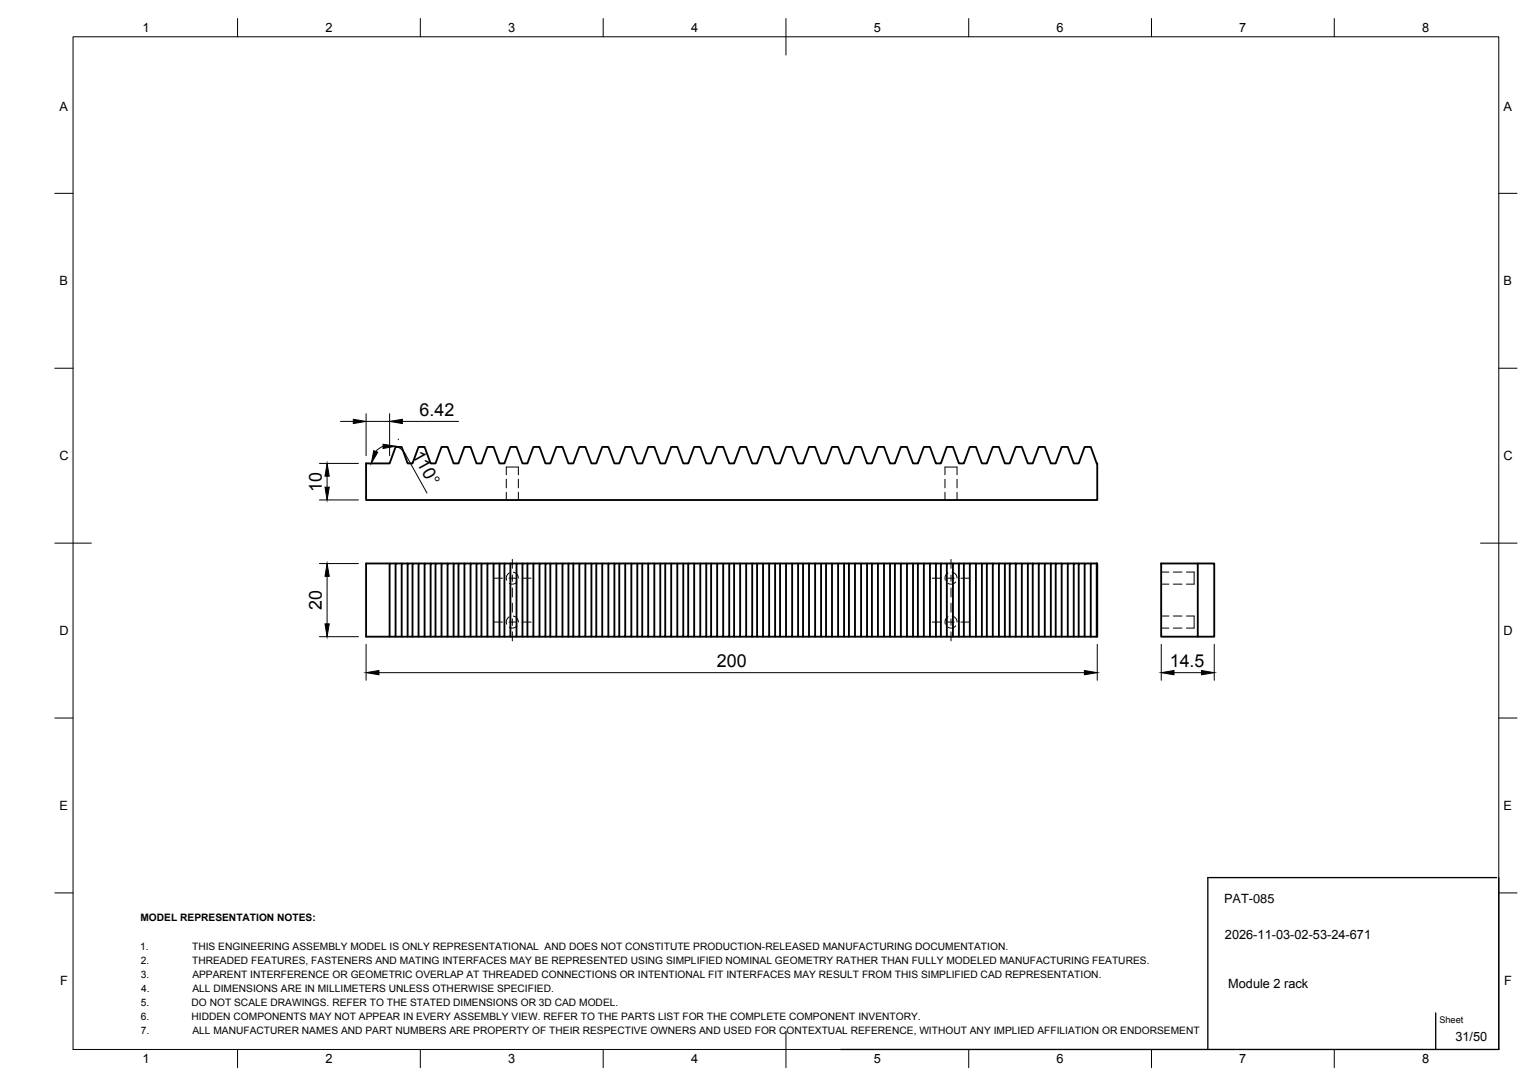
ISO-10303-21;
HEADER;
/* Generated by software containing ST-Developer
 * from STEP Tools, Inc. (www.steptools.com) 
 */

FILE_DESCRIPTION(
/* description */ ('Rack and pinion manual slide'),
/* implementation_level */ '2;1');

FILE_NAME(
/* name */ 'Module 2 rack.step',
/* time_stamp */ '2026-10-28T03:22:49-07:00',
/* author */ (''),
/* organization */ (''),
/* preprocessor_version */ 'ST-DEVELOPER v20.2',
/* originating_system */ 'Autodesk Translation Framework v15.17.0.0',
/* authorisation */ '');

FILE_SCHEMA (('AUTOMOTIVE_DESIGN { 1 0 10303 214 3 1 1 }'));
ENDSEC;

DATA;
#10=MECHANICAL_DESIGN_GEOMETRIC_PRESENTATION_REPRESENTATION('',(#765),#34851);
#666=SHAPE_REPRESENTATION_RELATIONSHIP('SRR','None',#35103,#712);
#712=ADVANCED_BREP_SHAPE_REPRESENTATION('',(#816),#34828);
#765=STYLED_ITEM('',(#35397),#816);
#816=MANIFOLD_SOLID_BREP('Body1',#13787);
#1001=FACE_BOUND('',#2793,.T.);
#1002=FACE_BOUND('',#2794,.T.);
#1003=FACE_BOUND('',#2795,.T.);
#1004=FACE_BOUND('',#2796,.T.);
#1251=PLANE('',#14966);
#1252=PLANE('',#14970);
#1253=PLANE('',#14974);
#1254=PLANE('',#14978);
#1255=PLANE('',#14979);
#1256=PLANE('',#14980);
#1257=PLANE('',#14981);
#1258=PLANE('',#14982);
#1259=PLANE('',#14983);
#1260=PLANE('',#14984);
#1261=PLANE('',#14985);
#1262=PLANE('',#14986);
#1263=PLANE('',#14987);
#1264=PLANE('',#14988);
#1265=PLANE('',#14989);
#1266=PLANE('',#14990);
#1267=PLANE('',#14991);
#1268=PLANE('',#14992);
#1269=PLANE('',#14993);
#1270=PLANE('',#14994);
#1271=PLANE('',#14995);
#1272=PLANE('',#14996);
#1273=PLANE('',#14997);
#1274=PLANE('',#14998);
#1275=PLANE('',#14999);
#1276=PLANE('',#15000);
#1277=PLANE('',#15001);
#1278=PLANE('',#15002);
#1279=PLANE('',#15003);
#1280=PLANE('',#15004);
#1281=PLANE('',#15005);
#1282=PLANE('',#15006);
#1283=PLANE('',#15007);
#1284=PLANE('',#15008);
#1285=PLANE('',#15009);
#1286=PLANE('',#15010);
#1287=PLANE('',#15011);
#1288=PLANE('',#15012);
#1289=PLANE('',#15013);
#1290=PLANE('',#15014);
#1291=PLANE('',#15015);
#1292=PLANE('',#15016);
#1293=PLANE('',#15017);
#1294=PLANE('',#15018);
#1295=PLANE('',#15019);
#1296=PLANE('',#15020);
#1297=PLANE('',#15021);
#1298=PLANE('',#15022);
#1299=PLANE('',#15023);
#1300=PLANE('',#15024);
#1301=PLANE('',#15025);
#1302=PLANE('',#15026);
#1303=PLANE('',#15027);
#1304=PLANE('',#15028);
#1305=PLANE('',#15029);
#1306=PLANE('',#15030);
#1307=PLANE('',#15031);
#1308=PLANE('',#15032);
#1309=PLANE('',#15033);
#1310=PLANE('',#15034);
#1311=PLANE('',#15035);
#1312=PLANE('',#15036);
#1313=PLANE('',#15037);
#1314=PLANE('',#15038);
#1315=PLANE('',#15039);
#1316=PLANE('',#15040);
#1317=PLANE('',#15041);
#1318=PLANE('',#15042);
#1319=PLANE('',#15043);
#1320=PLANE('',#15044);
#1321=PLANE('',#15045);
#1322=PLANE('',#15046);
#1323=PLANE('',#15047);
#1324=PLANE('',#15048);
#1325=PLANE('',#15049);
#1326=PLANE('',#15050);
#1327=PLANE('',#15051);
#1328=PLANE('',#15052);
#1329=PLANE('',#15053);
#1330=PLANE('',#15054);
#1331=PLANE('',#15055);
#1332=PLANE('',#15056);
#1333=PLANE('',#15057);
#1334=PLANE('',#15058);
#1335=PLANE('',#15059);
#1336=PLANE('',#15060);
#1337=PLANE('',#15061);
#1338=PLANE('',#15062);
#1339=PLANE('',#15063);
#1340=PLANE('',#15064);
#1341=PLANE('',#15065);
#1342=PLANE('',#15066);
#1343=PLANE('',#15067);
#1344=PLANE('',#15068);
#1345=PLANE('',#15069);
#1346=PLANE('',#15070);
#1347=PLANE('',#15071);
#1348=PLANE('',#15072);
#1349=PLANE('',#15073);
#1350=PLANE('',#15074);
#1351=PLANE('',#15075);
#1352=PLANE('',#15076);
#1353=PLANE('',#15077);
#1354=PLANE('',#15078);
#1355=PLANE('',#15079);
#1356=PLANE('',#15080);
#1357=PLANE('',#15081);
#1358=PLANE('',#15082);
#1359=PLANE('',#15083);
#1360=PLANE('',#15084);
#1361=PLANE('',#15085);
#1362=PLANE('',#15086);
#1363=PLANE('',#15087);
#1364=PLANE('',#15088);
#1365=PLANE('',#15089);
#1366=PLANE('',#15090);
#1367=PLANE('',#15091);
#1368=PLANE('',#15092);
#1369=PLANE('',#15093);
#1370=PLANE('',#15094);
#1371=PLANE('',#15095);
#1372=PLANE('',#15096);
#1373=PLANE('',#15097);
#1374=PLANE('',#15098);
#1375=PLANE('',#15099);
#1376=PLANE('',#15100);
#1377=PLANE('',#15101);
#1378=PLANE('',#15102);
#1379=PLANE('',#15103);
#1380=PLANE('',#15104);
#1381=PLANE('',#15105);
#1382=PLANE('',#15106);
#1383=PLANE('',#15107);
#1384=PLANE('',#15108);
#1876=FACE_OUTER_BOUND('',#2783,.T.);
#1877=FACE_OUTER_BOUND('',#2784,.T.);
#1878=FACE_OUTER_BOUND('',#2785,.T.);
#1879=FACE_OUTER_BOUND('',#2786,.T.);
#1880=FACE_OUTER_BOUND('',#2787,.T.);
#1881=FACE_OUTER_BOUND('',#2788,.T.);
#1882=FACE_OUTER_BOUND('',#2789,.T.);
#1883=FACE_OUTER_BOUND('',#2790,.T.);
#1884=FACE_OUTER_BOUND('',#2791,.T.);
#1885=FACE_OUTER_BOUND('',#2792,.T.);
#1886=FACE_OUTER_BOUND('',#2797,.T.);
#1887=FACE_OUTER_BOUND('',#2798,.T.);
#1888=FACE_OUTER_BOUND('',#2799,.T.);
#1889=FACE_OUTER_BOUND('',#2800,.T.);
#1890=FACE_OUTER_BOUND('',#2801,.T.);
#1891=FACE_OUTER_BOUND('',#2802,.T.);
#1892=FACE_OUTER_BOUND('',#2803,.T.);
#1893=FACE_OUTER_BOUND('',#2804,.T.);
#1894=FACE_OUTER_BOUND('',#2805,.T.);
#1895=FACE_OUTER_BOUND('',#2806,.T.);
#1896=FACE_OUTER_BOUND('',#2807,.T.);
#1897=FACE_OUTER_BOUND('',#2808,.T.);
#1898=FACE_OUTER_BOUND('',#2809,.T.);
#1899=FACE_OUTER_BOUND('',#2810,.T.);
#1900=FACE_OUTER_BOUND('',#2811,.T.);
#1901=FACE_OUTER_BOUND('',#2812,.T.);
#1902=FACE_OUTER_BOUND('',#2813,.T.);
#1903=FACE_OUTER_BOUND('',#2814,.T.);
#1904=FACE_OUTER_BOUND('',#2815,.T.);
#1905=FACE_OUTER_BOUND('',#2816,.T.);
#1906=FACE_OUTER_BOUND('',#2817,.T.);
#1907=FACE_OUTER_BOUND('',#2818,.T.);
#1908=FACE_OUTER_BOUND('',#2819,.T.);
#1909=FACE_OUTER_BOUND('',#2820,.T.);
#1910=FACE_OUTER_BOUND('',#2821,.T.);
#1911=FACE_OUTER_BOUND('',#2822,.T.);
#1912=FACE_OUTER_BOUND('',#2823,.T.);
#1913=FACE_OUTER_BOUND('',#2824,.T.);
#1914=FACE_OUTER_BOUND('',#2825,.T.);
#1915=FACE_OUTER_BOUND('',#2826,.T.);
#1916=FACE_OUTER_BOUND('',#2827,.T.);
#1917=FACE_OUTER_BOUND('',#2828,.T.);
#1918=FACE_OUTER_BOUND('',#2829,.T.);
#1919=FACE_OUTER_BOUND('',#2830,.T.);
#1920=FACE_OUTER_BOUND('',#2831,.T.);
#1921=FACE_OUTER_BOUND('',#2832,.T.);
#1922=FACE_OUTER_BOUND('',#2833,.T.);
#1923=FACE_OUTER_BOUND('',#2834,.T.);
#1924=FACE_OUTER_BOUND('',#2835,.T.);
#1925=FACE_OUTER_BOUND('',#2836,.T.);
#1926=FACE_OUTER_BOUND('',#2837,.T.);
#1927=FACE_OUTER_BOUND('',#2838,.T.);
#1928=FACE_OUTER_BOUND('',#2839,.T.);
#1929=FACE_OUTER_BOUND('',#2840,.T.);
#1930=FACE_OUTER_BOUND('',#2841,.T.);
#1931=FACE_OUTER_BOUND('',#2842,.T.);
#1932=FACE_OUTER_BOUND('',#2843,.T.);
#1933=FACE_OUTER_BOUND('',#2844,.T.);
#1934=FACE_OUTER_BOUND('',#2845,.T.);
#1935=FACE_OUTER_BOUND('',#2846,.T.);
#1936=FACE_OUTER_BOUND('',#2847,.T.);
#1937=FACE_OUTER_BOUND('',#2848,.T.);
#1938=FACE_OUTER_BOUND('',#2849,.T.);
#1939=FACE_OUTER_BOUND('',#2850,.T.);
#1940=FACE_OUTER_BOUND('',#2851,.T.);
#1941=FACE_OUTER_BOUND('',#2852,.T.);
#1942=FACE_OUTER_BOUND('',#2853,.T.);
#1943=FACE_OUTER_BOUND('',#2854,.T.);
#1944=FACE_OUTER_BOUND('',#2855,.T.);
#1945=FACE_OUTER_BOUND('',#2856,.T.);
#1946=FACE_OUTER_BOUND('',#2857,.T.);
#1947=FACE_OUTER_BOUND('',#2858,.T.);
#1948=FACE_OUTER_BOUND('',#2859,.T.);
#1949=FACE_OUTER_BOUND('',#2860,.T.);
#1950=FACE_OUTER_BOUND('',#2861,.T.);
#1951=FACE_OUTER_BOUND('',#2862,.T.);
#1952=FACE_OUTER_BOUND('',#2863,.T.);
#1953=FACE_OUTER_BOUND('',#2864,.T.);
#1954=FACE_OUTER_BOUND('',#2865,.T.);
#1955=FACE_OUTER_BOUND('',#2866,.T.);
#1956=FACE_OUTER_BOUND('',#2867,.T.);
#1957=FACE_OUTER_BOUND('',#2868,.T.);
#1958=FACE_OUTER_BOUND('',#2869,.T.);
#1959=FACE_OUTER_BOUND('',#2870,.T.);
#1960=FACE_OUTER_BOUND('',#2871,.T.);
#1961=FACE_OUTER_BOUND('',#2872,.T.);
#1962=FACE_OUTER_BOUND('',#2873,.T.);
#1963=FACE_OUTER_BOUND('',#2874,.T.);
#1964=FACE_OUTER_BOUND('',#2875,.T.);
#1965=FACE_OUTER_BOUND('',#2876,.T.);
#1966=FACE_OUTER_BOUND('',#2877,.T.);
#1967=FACE_OUTER_BOUND('',#2878,.T.);
#1968=FACE_OUTER_BOUND('',#2879,.T.);
#1969=FACE_OUTER_BOUND('',#2880,.T.);
#1970=FACE_OUTER_BOUND('',#2881,.T.);
#1971=FACE_OUTER_BOUND('',#2882,.T.);
#1972=FACE_OUTER_BOUND('',#2883,.T.);
#1973=FACE_OUTER_BOUND('',#2884,.T.);
#1974=FACE_OUTER_BOUND('',#2885,.T.);
#1975=FACE_OUTER_BOUND('',#2886,.T.);
#1976=FACE_OUTER_BOUND('',#2887,.T.);
#1977=FACE_OUTER_BOUND('',#2888,.T.);
#1978=FACE_OUTER_BOUND('',#2889,.T.);
#1979=FACE_OUTER_BOUND('',#2890,.T.);
#1980=FACE_OUTER_BOUND('',#2891,.T.);
#1981=FACE_OUTER_BOUND('',#2892,.T.);
#1982=FACE_OUTER_BOUND('',#2893,.T.);
#1983=FACE_OUTER_BOUND('',#2894,.T.);
#1984=FACE_OUTER_BOUND('',#2895,.T.);
#1985=FACE_OUTER_BOUND('',#2896,.T.);
#1986=FACE_OUTER_BOUND('',#2897,.T.);
#1987=FACE_OUTER_BOUND('',#2898,.T.);
#1988=FACE_OUTER_BOUND('',#2899,.T.);
#1989=FACE_OUTER_BOUND('',#2900,.T.);
#1990=FACE_OUTER_BOUND('',#2901,.T.);
#1991=FACE_OUTER_BOUND('',#2902,.T.);
#1992=FACE_OUTER_BOUND('',#2903,.T.);
#1993=FACE_OUTER_BOUND('',#2904,.T.);
#1994=FACE_OUTER_BOUND('',#2905,.T.);
#1995=FACE_OUTER_BOUND('',#2906,.T.);
#1996=FACE_OUTER_BOUND('',#2907,.T.);
#1997=FACE_OUTER_BOUND('',#2908,.T.);
#1998=FACE_OUTER_BOUND('',#2909,.T.);
#1999=FACE_OUTER_BOUND('',#2910,.T.);
#2000=FACE_OUTER_BOUND('',#2911,.T.);
#2001=FACE_OUTER_BOUND('',#2912,.T.);
#2002=FACE_OUTER_BOUND('',#2913,.T.);
#2003=FACE_OUTER_BOUND('',#2914,.T.);
#2004=FACE_OUTER_BOUND('',#2915,.T.);
#2005=FACE_OUTER_BOUND('',#2916,.T.);
#2006=FACE_OUTER_BOUND('',#2917,.T.);
#2007=FACE_OUTER_BOUND('',#2918,.T.);
#2008=FACE_OUTER_BOUND('',#2919,.T.);
#2009=FACE_OUTER_BOUND('',#2920,.T.);
#2010=FACE_OUTER_BOUND('',#2921,.T.);
#2011=FACE_OUTER_BOUND('',#2922,.T.);
#2012=FACE_OUTER_BOUND('',#2923,.T.);
#2013=FACE_OUTER_BOUND('',#2924,.T.);
#2783=EDGE_LOOP('',(#10820,#10821,#10822,#10823));
#2784=EDGE_LOOP('',(#10824));
#2785=EDGE_LOOP('',(#10825,#10826,#10827,#10828));
#2786=EDGE_LOOP('',(#10829));
#2787=EDGE_LOOP('',(#10830,#10831,#10832,#10833));
#2788=EDGE_LOOP('',(#10834));
#2789=EDGE_LOOP('',(#10835,#10836,#10837,#10838));
#2790=EDGE_LOOP('',(#10839));
#2791=EDGE_LOOP('',(#10840,#10841,#10842,#10843));
#2792=EDGE_LOOP('',(#10844,#10845,#10846,#10847));
#2793=EDGE_LOOP('',(#10848));
#2794=EDGE_LOOP('',(#10849));
#2795=EDGE_LOOP('',(#10850));
#2796=EDGE_LOOP('',(#10851));
#2797=EDGE_LOOP('',(#10852,#10853,#10854,#10855));
#2798=EDGE_LOOP('',(#10856,#10857,#10858,#10859));
#2799=EDGE_LOOP('',(#10860,#10861,#10862,#10863));
#2800=EDGE_LOOP('',(#10864,#10865,#10866,#10867));
#2801=EDGE_LOOP('',(#10868,#10869,#10870,#10871));
#2802=EDGE_LOOP('',(#10872,#10873,#10874,#10875));
#2803=EDGE_LOOP('',(#10876,#10877,#10878,#10879));
#2804=EDGE_LOOP('',(#10880,#10881,#10882,#10883));
#2805=EDGE_LOOP('',(#10884,#10885,#10886,#10887));
#2806=EDGE_LOOP('',(#10888,#10889,#10890,#10891));
#2807=EDGE_LOOP('',(#10892,#10893,#10894,#10895));
#2808=EDGE_LOOP('',(#10896,#10897,#10898,#10899));
#2809=EDGE_LOOP('',(#10900,#10901,#10902,#10903));
#2810=EDGE_LOOP('',(#10904,#10905,#10906,#10907));
#2811=EDGE_LOOP('',(#10908,#10909,#10910,#10911));
#2812=EDGE_LOOP('',(#10912,#10913,#10914,#10915));
#2813=EDGE_LOOP('',(#10916,#10917,#10918,#10919));
#2814=EDGE_LOOP('',(#10920,#10921,#10922,#10923));
#2815=EDGE_LOOP('',(#10924,#10925,#10926,#10927));
#2816=EDGE_LOOP('',(#10928,#10929,#10930,#10931));
#2817=EDGE_LOOP('',(#10932,#10933,#10934,#10935));
#2818=EDGE_LOOP('',(#10936,#10937,#10938,#10939));
#2819=EDGE_LOOP('',(#10940,#10941,#10942,#10943));
#2820=EDGE_LOOP('',(#10944,#10945,#10946,#10947));
#2821=EDGE_LOOP('',(#10948,#10949,#10950,#10951));
#2822=EDGE_LOOP('',(#10952,#10953,#10954,#10955));
#2823=EDGE_LOOP('',(#10956,#10957,#10958,#10959));
#2824=EDGE_LOOP('',(#10960,#10961,#10962,#10963));
#2825=EDGE_LOOP('',(#10964,#10965,#10966,#10967));
#2826=EDGE_LOOP('',(#10968,#10969,#10970,#10971));
#2827=EDGE_LOOP('',(#10972,#10973,#10974,#10975));
#2828=EDGE_LOOP('',(#10976,#10977,#10978,#10979));
#2829=EDGE_LOOP('',(#10980,#10981,#10982,#10983));
#2830=EDGE_LOOP('',(#10984,#10985,#10986,#10987));
#2831=EDGE_LOOP('',(#10988,#10989,#10990,#10991));
#2832=EDGE_LOOP('',(#10992,#10993,#10994,#10995));
#2833=EDGE_LOOP('',(#10996,#10997,#10998,#10999));
#2834=EDGE_LOOP('',(#11000,#11001,#11002,#11003));
#2835=EDGE_LOOP('',(#11004,#11005,#11006,#11007));
#2836=EDGE_LOOP('',(#11008,#11009,#11010,#11011));
#2837=EDGE_LOOP('',(#11012,#11013,#11014,#11015));
#2838=EDGE_LOOP('',(#11016,#11017,#11018,#11019));
#2839=EDGE_LOOP('',(#11020,#11021,#11022,#11023));
#2840=EDGE_LOOP('',(#11024,#11025,#11026,#11027));
#2841=EDGE_LOOP('',(#11028,#11029,#11030,#11031));
#2842=EDGE_LOOP('',(#11032,#11033,#11034,#11035));
#2843=EDGE_LOOP('',(#11036,#11037,#11038,#11039));
#2844=EDGE_LOOP('',(#11040,#11041,#11042,#11043));
#2845=EDGE_LOOP('',(#11044,#11045,#11046,#11047));
#2846=EDGE_LOOP('',(#11048,#11049,#11050,#11051));
#2847=EDGE_LOOP('',(#11052,#11053,#11054,#11055));
#2848=EDGE_LOOP('',(#11056,#11057,#11058,#11059));
#2849=EDGE_LOOP('',(#11060,#11061,#11062,#11063));
#2850=EDGE_LOOP('',(#11064,#11065,#11066,#11067));
#2851=EDGE_LOOP('',(#11068,#11069,#11070,#11071));
#2852=EDGE_LOOP('',(#11072,#11073,#11074,#11075));
#2853=EDGE_LOOP('',(#11076,#11077,#11078,#11079));
#2854=EDGE_LOOP('',(#11080,#11081,#11082,#11083));
#2855=EDGE_LOOP('',(#11084,#11085,#11086,#11087));
#2856=EDGE_LOOP('',(#11088,#11089,#11090,#11091));
#2857=EDGE_LOOP('',(#11092,#11093,#11094,#11095));
#2858=EDGE_LOOP('',(#11096,#11097,#11098,#11099));
#2859=EDGE_LOOP('',(#11100,#11101,#11102,#11103));
#2860=EDGE_LOOP('',(#11104,#11105,#11106,#11107));
#2861=EDGE_LOOP('',(#11108,#11109,#11110,#11111));
#2862=EDGE_LOOP('',(#11112,#11113,#11114,#11115));
#2863=EDGE_LOOP('',(#11116,#11117,#11118,#11119));
#2864=EDGE_LOOP('',(#11120,#11121,#11122,#11123));
#2865=EDGE_LOOP('',(#11124,#11125,#11126,#11127));
#2866=EDGE_LOOP('',(#11128,#11129,#11130,#11131));
#2867=EDGE_LOOP('',(#11132,#11133,#11134,#11135));
#2868=EDGE_LOOP('',(#11136,#11137,#11138,#11139));
#2869=EDGE_LOOP('',(#11140,#11141,#11142,#11143));
#2870=EDGE_LOOP('',(#11144,#11145,#11146,#11147));
#2871=EDGE_LOOP('',(#11148,#11149,#11150,#11151));
#2872=EDGE_LOOP('',(#11152,#11153,#11154,#11155));
#2873=EDGE_LOOP('',(#11156,#11157,#11158,#11159));
#2874=EDGE_LOOP('',(#11160,#11161,#11162,#11163));
#2875=EDGE_LOOP('',(#11164,#11165,#11166,#11167));
#2876=EDGE_LOOP('',(#11168,#11169,#11170,#11171));
#2877=EDGE_LOOP('',(#11172,#11173,#11174,#11175));
#2878=EDGE_LOOP('',(#11176,#11177,#11178,#11179));
#2879=EDGE_LOOP('',(#11180,#11181,#11182,#11183));
#2880=EDGE_LOOP('',(#11184,#11185,#11186,#11187));
#2881=EDGE_LOOP('',(#11188,#11189,#11190,#11191));
#2882=EDGE_LOOP('',(#11192,#11193,#11194,#11195));
#2883=EDGE_LOOP('',(#11196,#11197,#11198,#11199));
#2884=EDGE_LOOP('',(#11200,#11201,#11202,#11203));
#2885=EDGE_LOOP('',(#11204,#11205,#11206,#11207));
#2886=EDGE_LOOP('',(#11208,#11209,#11210,#11211));
#2887=EDGE_LOOP('',(#11212,#11213,#11214,#11215));
#2888=EDGE_LOOP('',(#11216,#11217,#11218,#11219));
#2889=EDGE_LOOP('',(#11220,#11221,#11222,#11223));
#2890=EDGE_LOOP('',(#11224,#11225,#11226,#11227));
#2891=EDGE_LOOP('',(#11228,#11229,#11230,#11231));
#2892=EDGE_LOOP('',(#11232,#11233,#11234,#11235));
#2893=EDGE_LOOP('',(#11236,#11237,#11238,#11239));
#2894=EDGE_LOOP('',(#11240,#11241,#11242,#11243));
#2895=EDGE_LOOP('',(#11244,#11245,#11246,#11247));
#2896=EDGE_LOOP('',(#11248,#11249,#11250,#11251));
#2897=EDGE_LOOP('',(#11252,#11253,#11254,#11255));
#2898=EDGE_LOOP('',(#11256,#11257,#11258,#11259));
#2899=EDGE_LOOP('',(#11260,#11261,#11262,#11263));
#2900=EDGE_LOOP('',(#11264,#11265,#11266,#11267));
#2901=EDGE_LOOP('',(#11268,#11269,#11270,#11271));
#2902=EDGE_LOOP('',(#11272,#11273,#11274,#11275));
#2903=EDGE_LOOP('',(#11276,#11277,#11278,#11279));
#2904=EDGE_LOOP('',(#11280,#11281,#11282,#11283));
#2905=EDGE_LOOP('',(#11284,#11285,#11286,#11287));
#2906=EDGE_LOOP('',(#11288,#11289,#11290,#11291));
#2907=EDGE_LOOP('',(#11292,#11293,#11294,#11295));
#2908=EDGE_LOOP('',(#11296,#11297,#11298,#11299));
#2909=EDGE_LOOP('',(#11300,#11301,#11302,#11303));
#2910=EDGE_LOOP('',(#11304,#11305,#11306,#11307));
#2911=EDGE_LOOP('',(#11308,#11309,#11310,#11311));
#2912=EDGE_LOOP('',(#11312,#11313,#11314,#11315));
#2913=EDGE_LOOP('',(#11316,#11317,#11318,#11319));
#2914=EDGE_LOOP('',(#11320,#11321,#11322,#11323));
#2915=EDGE_LOOP('',(#11324,#11325,#11326,#11327));
#2916=EDGE_LOOP('',(#11328,#11329,#11330,#11331));
#2917=EDGE_LOOP('',(#11332,#11333,#11334,#11335));
#2918=EDGE_LOOP('',(#11336,#11337,#11338,#11339));
#2919=EDGE_LOOP('',(#11340,#11341,#11342,#11343));
#2920=EDGE_LOOP('',(#11344,#11345,#11346,#11347));
#2921=EDGE_LOOP('',(#11348,#11349,#11350,#11351));
#2922=EDGE_LOOP('',(#11352,#11353,#11354,#11355));
#2923=EDGE_LOOP('',(#11356,#11357,#11358,#11359,#11360,#11361,#11362,#11363,
#11364,#11365,#11366,#11367,#11368,#11369,#11370,#11371,#11372,#11373,#11374,
#11375,#11376,#11377,#11378,#11379,#11380,#11381,#11382,#11383,#11384,#11385,
#11386,#11387,#11388,#11389,#11390,#11391,#11392,#11393,#11394,#11395,#11396,
#11397,#11398,#11399,#11400,#11401,#11402,#11403,#11404,#11405,#11406,#11407,
#11408,#11409,#11410,#11411,#11412,#11413,#11414,#11415,#11416,#11417,#11418,
#11419,#11420,#11421,#11422,#11423,#11424,#11425,#11426,#11427,#11428,#11429,
#11430,#11431,#11432,#11433,#11434,#11435,#11436,#11437,#11438,#11439,#11440,
#11441,#11442,#11443,#11444,#11445,#11446,#11447,#11448,#11449,#11450,#11451,
#11452,#11453,#11454,#11455,#11456,#11457,#11458,#11459,#11460,#11461,#11462,
#11463,#11464,#11465,#11466,#11467,#11468,#11469,#11470,#11471,#11472,#11473,
#11474,#11475,#11476,#11477,#11478,#11479,#11480,#11481,#11482,#11483));
#2924=EDGE_LOOP('',(#11484,#11485,#11486,#11487,#11488,#11489,#11490,#11491,
#11492,#11493,#11494,#11495,#11496,#11497,#11498,#11499,#11500,#11501,#11502,
#11503,#11504,#11505,#11506,#11507,#11508,#11509,#11510,#11511,#11512,#11513,
#11514,#11515,#11516,#11517,#11518,#11519,#11520,#11521,#11522,#11523,#11524,
#11525,#11526,#11527,#11528,#11529,#11530,#11531,#11532,#11533,#11534,#11535,
#11536,#11537,#11538,#11539,#11540,#11541,#11542,#11543,#11544,#11545,#11546,
#11547,#11548,#11549,#11550,#11551,#11552,#11553,#11554,#11555,#11556,#11557,
#11558,#11559,#11560,#11561,#11562,#11563,#11564,#11565,#11566,#11567,#11568,
#11569,#11570,#11571,#11572,#11573,#11574,#11575,#11576,#11577,#11578,#11579,
#11580,#11581,#11582,#11583,#11584,#11585,#11586,#11587,#11588,#11589,#11590,
#11591,#11592,#11593,#11594,#11595,#11596,#11597,#11598,#11599,#11600,#11601,
#11602,#11603,#11604,#11605,#11606,#11607,#11608,#11609,#11610,#11611));
#3734=LINE('',#21459,#5025);
#3735=LINE('',#21466,#5026);
#3736=LINE('',#21473,#5027);
#3737=LINE('',#21480,#5028);
#3738=LINE('',#21486,#5029);
#3739=LINE('',#21488,#5030);
#3740=LINE('',#21490,#5031);
#3741=LINE('',#21491,#5032);
#3742=LINE('',#21494,#5033);
#3743=LINE('',#21496,#5034);
#3744=LINE('',#21497,#5035);
#3745=LINE('',#21500,#5036);
#3746=LINE('',#21502,#5037);
#3747=LINE('',#21503,#5038);
#3748=LINE('',#21506,#5039);
#3749=LINE('',#21508,#5040);
#3750=LINE('',#21509,#5041);
#3751=LINE('',#21512,#5042);
#3752=LINE('',#21514,#5043);
#3753=LINE('',#21515,#5044);
#3754=LINE('',#21518,#5045);
#3755=LINE('',#21520,#5046);
#3756=LINE('',#21521,#5047);
#3757=LINE('',#21524,#5048);
#3758=LINE('',#21526,#5049);
#3759=LINE('',#21527,#5050);
#3760=LINE('',#21530,#5051);
#3761=LINE('',#21532,#5052);
#3762=LINE('',#21533,#5053);
#3763=LINE('',#21536,#5054);
#3764=LINE('',#21538,#5055);
#3765=LINE('',#21539,#5056);
#3766=LINE('',#21542,#5057);
#3767=LINE('',#21544,#5058);
#3768=LINE('',#21545,#5059);
#3769=LINE('',#21548,#5060);
#3770=LINE('',#21550,#5061);
#3771=LINE('',#21551,#5062);
#3772=LINE('',#21554,#5063);
#3773=LINE('',#21556,#5064);
#3774=LINE('',#21557,#5065);
#3775=LINE('',#21560,#5066);
#3776=LINE('',#21562,#5067);
#3777=LINE('',#21563,#5068);
#3778=LINE('',#21566,#5069);
#3779=LINE('',#21568,#5070);
#3780=LINE('',#21569,#5071);
#3781=LINE('',#21572,#5072);
#3782=LINE('',#21574,#5073);
#3783=LINE('',#21575,#5074);
#3784=LINE('',#21578,#5075);
#3785=LINE('',#21580,#5076);
#3786=LINE('',#21581,#5077);
#3787=LINE('',#21584,#5078);
#3788=LINE('',#21586,#5079);
#3789=LINE('',#21587,#5080);
#3790=LINE('',#21590,#5081);
#3791=LINE('',#21592,#5082);
#3792=LINE('',#21593,#5083);
#3793=LINE('',#21596,#5084);
#3794=LINE('',#21598,#5085);
#3795=LINE('',#21599,#5086);
#3796=LINE('',#21602,#5087);
#3797=LINE('',#21604,#5088);
#3798=LINE('',#21605,#5089);
#3799=LINE('',#21608,#5090);
#3800=LINE('',#21610,#5091);
#3801=LINE('',#21611,#5092);
#3802=LINE('',#21614,#5093);
#3803=LINE('',#21616,#5094);
#3804=LINE('',#21617,#5095);
#3805=LINE('',#21620,#5096);
#3806=LINE('',#21622,#5097);
#3807=LINE('',#21623,#5098);
#3808=LINE('',#21626,#5099);
#3809=LINE('',#21628,#5100);
#3810=LINE('',#21629,#5101);
#3811=LINE('',#21632,#5102);
#3812=LINE('',#21634,#5103);
#3813=LINE('',#21635,#5104);
#3814=LINE('',#21638,#5105);
#3815=LINE('',#21640,#5106);
#3816=LINE('',#21641,#5107);
#3817=LINE('',#21644,#5108);
#3818=LINE('',#21646,#5109);
#3819=LINE('',#21647,#5110);
#3820=LINE('',#21650,#5111);
#3821=LINE('',#21652,#5112);
#3822=LINE('',#21653,#5113);
#3823=LINE('',#21656,#5114);
#3824=LINE('',#21658,#5115);
#3825=LINE('',#21659,#5116);
#3826=LINE('',#21662,#5117);
#3827=LINE('',#21664,#5118);
#3828=LINE('',#21665,#5119);
#3829=LINE('',#21668,#5120);
#3830=LINE('',#21670,#5121);
#3831=LINE('',#21671,#5122);
#3832=LINE('',#21674,#5123);
#3833=LINE('',#21676,#5124);
#3834=LINE('',#21677,#5125);
#3835=LINE('',#21680,#5126);
#3836=LINE('',#21682,#5127);
#3837=LINE('',#21683,#5128);
#3838=LINE('',#21686,#5129);
#3839=LINE('',#21688,#5130);
#3840=LINE('',#21689,#5131);
#3841=LINE('',#21692,#5132);
#3842=LINE('',#21694,#5133);
#3843=LINE('',#21695,#5134);
#3844=LINE('',#21698,#5135);
#3845=LINE('',#21700,#5136);
#3846=LINE('',#21701,#5137);
#3847=LINE('',#21704,#5138);
#3848=LINE('',#21706,#5139);
#3849=LINE('',#21707,#5140);
#3850=LINE('',#21710,#5141);
#3851=LINE('',#21712,#5142);
#3852=LINE('',#21713,#5143);
#3853=LINE('',#21716,#5144);
#3854=LINE('',#21718,#5145);
#3855=LINE('',#21719,#5146);
#3856=LINE('',#21722,#5147);
#3857=LINE('',#21724,#5148);
#3858=LINE('',#21725,#5149);
#3859=LINE('',#21728,#5150);
#3860=LINE('',#21730,#5151);
#3861=LINE('',#21731,#5152);
#3862=LINE('',#21734,#5153);
#3863=LINE('',#21736,#5154);
#3864=LINE('',#21737,#5155);
#3865=LINE('',#21740,#5156);
#3866=LINE('',#21742,#5157);
#3867=LINE('',#21743,#5158);
#3868=LINE('',#21746,#5159);
#3869=LINE('',#21748,#5160);
#3870=LINE('',#21749,#5161);
#3871=LINE('',#21752,#5162);
#3872=LINE('',#21754,#5163);
#3873=LINE('',#21755,#5164);
#3874=LINE('',#21758,#5165);
#3875=LINE('',#21760,#5166);
#3876=LINE('',#21761,#5167);
#3877=LINE('',#21764,#5168);
#3878=LINE('',#21766,#5169);
#3879=LINE('',#21767,#5170);
#3880=LINE('',#21770,#5171);
#3881=LINE('',#21772,#5172);
#3882=LINE('',#21773,#5173);
#3883=LINE('',#21776,#5174);
#3884=LINE('',#21778,#5175);
#3885=LINE('',#21779,#5176);
#3886=LINE('',#21782,#5177);
#3887=LINE('',#21784,#5178);
#3888=LINE('',#21785,#5179);
#3889=LINE('',#21788,#5180);
#3890=LINE('',#21790,#5181);
#3891=LINE('',#21791,#5182);
#3892=LINE('',#21794,#5183);
#3893=LINE('',#21796,#5184);
#3894=LINE('',#21797,#5185);
#3895=LINE('',#21800,#5186);
#3896=LINE('',#21802,#5187);
#3897=LINE('',#21803,#5188);
#3898=LINE('',#21806,#5189);
#3899=LINE('',#21808,#5190);
#3900=LINE('',#21809,#5191);
#3901=LINE('',#21812,#5192);
#3902=LINE('',#21814,#5193);
#3903=LINE('',#21815,#5194);
#3904=LINE('',#21818,#5195);
#3905=LINE('',#21820,#5196);
#3906=LINE('',#21821,#5197);
#3907=LINE('',#21824,#5198);
#3908=LINE('',#21826,#5199);
#3909=LINE('',#21827,#5200);
#3910=LINE('',#21830,#5201);
#3911=LINE('',#21832,#5202);
#3912=LINE('',#21833,#5203);
#3913=LINE('',#21836,#5204);
#3914=LINE('',#21838,#5205);
#3915=LINE('',#21839,#5206);
#3916=LINE('',#21842,#5207);
#3917=LINE('',#21844,#5208);
#3918=LINE('',#21845,#5209);
#3919=LINE('',#21848,#5210);
#3920=LINE('',#21850,#5211);
#3921=LINE('',#21851,#5212);
#3922=LINE('',#21854,#5213);
#3923=LINE('',#21856,#5214);
#3924=LINE('',#21857,#5215);
#3925=LINE('',#21860,#5216);
#3926=LINE('',#21862,#5217);
#3927=LINE('',#21863,#5218);
#3928=LINE('',#21866,#5219);
#3929=LINE('',#21868,#5220);
#3930=LINE('',#21869,#5221);
#3931=LINE('',#21872,#5222);
#3932=LINE('',#21874,#5223);
#3933=LINE('',#21875,#5224);
#3934=LINE('',#21878,#5225);
#3935=LINE('',#21880,#5226);
#3936=LINE('',#21881,#5227);
#3937=LINE('',#21884,#5228);
#3938=LINE('',#21886,#5229);
#3939=LINE('',#21887,#5230);
#3940=LINE('',#21890,#5231);
#3941=LINE('',#21892,#5232);
#3942=LINE('',#21893,#5233);
#3943=LINE('',#21896,#5234);
#3944=LINE('',#21898,#5235);
#3945=LINE('',#21899,#5236);
#3946=LINE('',#21902,#5237);
#3947=LINE('',#21904,#5238);
#3948=LINE('',#21905,#5239);
#3949=LINE('',#21908,#5240);
#3950=LINE('',#21910,#5241);
#3951=LINE('',#21911,#5242);
#3952=LINE('',#21914,#5243);
#3953=LINE('',#21916,#5244);
#3954=LINE('',#21917,#5245);
#3955=LINE('',#21920,#5246);
#3956=LINE('',#21922,#5247);
#3957=LINE('',#21923,#5248);
#3958=LINE('',#21926,#5249);
#3959=LINE('',#21928,#5250);
#3960=LINE('',#21929,#5251);
#3961=LINE('',#21932,#5252);
#3962=LINE('',#21934,#5253);
#3963=LINE('',#21935,#5254);
#3964=LINE('',#21938,#5255);
#3965=LINE('',#21940,#5256);
#3966=LINE('',#21941,#5257);
#3967=LINE('',#21944,#5258);
#3968=LINE('',#21946,#5259);
#3969=LINE('',#21947,#5260);
#3970=LINE('',#21950,#5261);
#3971=LINE('',#21952,#5262);
#3972=LINE('',#21953,#5263);
#3973=LINE('',#21956,#5264);
#3974=LINE('',#21958,#5265);
#3975=LINE('',#21959,#5266);
#3976=LINE('',#21962,#5267);
#3977=LINE('',#21964,#5268);
#3978=LINE('',#21965,#5269);
#3979=LINE('',#21968,#5270);
#3980=LINE('',#21970,#5271);
#3981=LINE('',#21971,#5272);
#3982=LINE('',#21974,#5273);
#3983=LINE('',#21976,#5274);
#3984=LINE('',#21977,#5275);
#3985=LINE('',#21980,#5276);
#3986=LINE('',#21982,#5277);
#3987=LINE('',#21983,#5278);
#3988=LINE('',#21986,#5279);
#3989=LINE('',#21988,#5280);
#3990=LINE('',#21989,#5281);
#3991=LINE('',#21992,#5282);
#3992=LINE('',#21994,#5283);
#3993=LINE('',#21995,#5284);
#3994=LINE('',#21998,#5285);
#3995=LINE('',#22000,#5286);
#3996=LINE('',#22001,#5287);
#3997=LINE('',#22004,#5288);
#3998=LINE('',#22006,#5289);
#3999=LINE('',#22007,#5290);
#4000=LINE('',#22010,#5291);
#4001=LINE('',#22012,#5292);
#4002=LINE('',#22013,#5293);
#4003=LINE('',#22016,#5294);
#4004=LINE('',#22018,#5295);
#4005=LINE('',#22019,#5296);
#4006=LINE('',#22022,#5297);
#4007=LINE('',#22024,#5298);
#4008=LINE('',#22025,#5299);
#4009=LINE('',#22028,#5300);
#4010=LINE('',#22030,#5301);
#4011=LINE('',#22031,#5302);
#4012=LINE('',#22034,#5303);
#4013=LINE('',#22036,#5304);
#4014=LINE('',#22037,#5305);
#4015=LINE('',#22040,#5306);
#4016=LINE('',#22042,#5307);
#4017=LINE('',#22043,#5308);
#4018=LINE('',#22046,#5309);
#4019=LINE('',#22048,#5310);
#4020=LINE('',#22049,#5311);
#4021=LINE('',#22052,#5312);
#4022=LINE('',#22054,#5313);
#4023=LINE('',#22055,#5314);
#4024=LINE('',#22058,#5315);
#4025=LINE('',#22060,#5316);
#4026=LINE('',#22061,#5317);
#4027=LINE('',#22064,#5318);
#4028=LINE('',#22066,#5319);
#4029=LINE('',#22067,#5320);
#4030=LINE('',#22070,#5321);
#4031=LINE('',#22072,#5322);
#4032=LINE('',#22073,#5323);
#4033=LINE('',#22076,#5324);
#4034=LINE('',#22078,#5325);
#4035=LINE('',#22079,#5326);
#4036=LINE('',#22082,#5327);
#4037=LINE('',#22084,#5328);
#4038=LINE('',#22085,#5329);
#4039=LINE('',#22088,#5330);
#4040=LINE('',#22090,#5331);
#4041=LINE('',#22091,#5332);
#4042=LINE('',#22094,#5333);
#4043=LINE('',#22096,#5334);
#4044=LINE('',#22097,#5335);
#4045=LINE('',#22100,#5336);
#4046=LINE('',#22102,#5337);
#4047=LINE('',#22103,#5338);
#4048=LINE('',#22106,#5339);
#4049=LINE('',#22108,#5340);
#4050=LINE('',#22109,#5341);
#4051=LINE('',#22112,#5342);
#4052=LINE('',#22114,#5343);
#4053=LINE('',#22115,#5344);
#4054=LINE('',#22118,#5345);
#4055=LINE('',#22120,#5346);
#4056=LINE('',#22121,#5347);
#4057=LINE('',#22124,#5348);
#4058=LINE('',#22126,#5349);
#4059=LINE('',#22127,#5350);
#4060=LINE('',#22130,#5351);
#4061=LINE('',#22132,#5352);
#4062=LINE('',#22133,#5353);
#4063=LINE('',#22136,#5354);
#4064=LINE('',#22138,#5355);
#4065=LINE('',#22139,#5356);
#4066=LINE('',#22142,#5357);
#4067=LINE('',#22144,#5358);
#4068=LINE('',#22145,#5359);
#4069=LINE('',#22148,#5360);
#4070=LINE('',#22150,#5361);
#4071=LINE('',#22151,#5362);
#4072=LINE('',#22154,#5363);
#4073=LINE('',#22156,#5364);
#4074=LINE('',#22157,#5365);
#4075=LINE('',#22160,#5366);
#4076=LINE('',#22162,#5367);
#4077=LINE('',#22163,#5368);
#4078=LINE('',#22166,#5369);
#4079=LINE('',#22168,#5370);
#4080=LINE('',#22169,#5371);
#4081=LINE('',#22172,#5372);
#4082=LINE('',#22174,#5373);
#4083=LINE('',#22175,#5374);
#4084=LINE('',#22178,#5375);
#4085=LINE('',#22180,#5376);
#4086=LINE('',#22181,#5377);
#4087=LINE('',#22184,#5378);
#4088=LINE('',#22186,#5379);
#4089=LINE('',#22187,#5380);
#4090=LINE('',#22190,#5381);
#4091=LINE('',#22192,#5382);
#4092=LINE('',#22193,#5383);
#4093=LINE('',#22196,#5384);
#4094=LINE('',#22198,#5385);
#4095=LINE('',#22199,#5386);
#4096=LINE('',#22202,#5387);
#4097=LINE('',#22204,#5388);
#4098=LINE('',#22205,#5389);
#4099=LINE('',#22208,#5390);
#4100=LINE('',#22210,#5391);
#4101=LINE('',#22211,#5392);
#4102=LINE('',#22214,#5393);
#4103=LINE('',#22216,#5394);
#4104=LINE('',#22217,#5395);
#4105=LINE('',#22220,#5396);
#4106=LINE('',#22222,#5397);
#4107=LINE('',#22223,#5398);
#4108=LINE('',#22226,#5399);
#4109=LINE('',#22228,#5400);
#4110=LINE('',#22229,#5401);
#4111=LINE('',#22232,#5402);
#4112=LINE('',#22234,#5403);
#4113=LINE('',#22235,#5404);
#4114=LINE('',#22238,#5405);
#4115=LINE('',#22240,#5406);
#4116=LINE('',#22241,#5407);
#4117=LINE('',#22244,#5408);
#4118=LINE('',#22246,#5409);
#4119=LINE('',#22247,#5410);
#4120=LINE('',#22249,#5411);
#4121=LINE('',#22250,#5412);
#5025=VECTOR('',#17406,0.164999999999999);
#5026=VECTOR('',#17415,0.165);
#5027=VECTOR('',#17424,0.165);
#5028=VECTOR('',#17433,0.164999999999999);
#5029=VECTOR('',#17440,1.);
#5030=VECTOR('',#17441,1.);
#5031=VECTOR('',#17442,1.);
#5032=VECTOR('',#17443,1.);
#5033=VECTOR('',#17446,1.);
#5034=VECTOR('',#17447,1.);
#5035=VECTOR('',#17448,1.);
#5036=VECTOR('',#17451,1.);
#5037=VECTOR('',#17452,1.);
#5038=VECTOR('',#17453,1.);
#5039=VECTOR('',#17456,1.);
#5040=VECTOR('',#17457,1.);
#5041=VECTOR('',#17458,1.);
#5042=VECTOR('',#17461,1.);
#5043=VECTOR('',#17462,1.);
#5044=VECTOR('',#17463,1.);
#5045=VECTOR('',#17466,1.);
#5046=VECTOR('',#17467,1.);
#5047=VECTOR('',#17468,1.);
#5048=VECTOR('',#17471,1.);
#5049=VECTOR('',#17472,1.);
#5050=VECTOR('',#17473,1.);
#5051=VECTOR('',#17476,1.);
#5052=VECTOR('',#17477,1.);
#5053=VECTOR('',#17478,1.);
#5054=VECTOR('',#17481,1.);
#5055=VECTOR('',#17482,1.);
#5056=VECTOR('',#17483,1.);
#5057=VECTOR('',#17486,1.);
#5058=VECTOR('',#17487,1.);
#5059=VECTOR('',#17488,1.);
#5060=VECTOR('',#17491,1.);
#5061=VECTOR('',#17492,1.);
#5062=VECTOR('',#17493,1.);
#5063=VECTOR('',#17496,1.);
#5064=VECTOR('',#17497,1.);
#5065=VECTOR('',#17498,1.);
#5066=VECTOR('',#17501,1.);
#5067=VECTOR('',#17502,1.);
#5068=VECTOR('',#17503,1.);
#5069=VECTOR('',#17506,1.);
#5070=VECTOR('',#17507,1.);
#5071=VECTOR('',#17508,1.);
#5072=VECTOR('',#17511,1.);
#5073=VECTOR('',#17512,1.);
#5074=VECTOR('',#17513,1.);
#5075=VECTOR('',#17516,1.);
#5076=VECTOR('',#17517,1.);
#5077=VECTOR('',#17518,1.);
#5078=VECTOR('',#17521,1.);
#5079=VECTOR('',#17522,1.);
#5080=VECTOR('',#17523,1.);
#5081=VECTOR('',#17526,1.);
#5082=VECTOR('',#17527,1.);
#5083=VECTOR('',#17528,1.);
#5084=VECTOR('',#17531,1.);
#5085=VECTOR('',#17532,1.);
#5086=VECTOR('',#17533,1.);
#5087=VECTOR('',#17536,1.);
#5088=VECTOR('',#17537,1.);
#5089=VECTOR('',#17538,1.);
#5090=VECTOR('',#17541,1.);
#5091=VECTOR('',#17542,1.);
#5092=VECTOR('',#17543,1.);
#5093=VECTOR('',#17546,1.);
#5094=VECTOR('',#17547,1.);
#5095=VECTOR('',#17548,1.);
#5096=VECTOR('',#17551,1.);
#5097=VECTOR('',#17552,1.);
#5098=VECTOR('',#17553,1.);
#5099=VECTOR('',#17556,1.);
#5100=VECTOR('',#17557,1.);
#5101=VECTOR('',#17558,1.);
#5102=VECTOR('',#17561,1.);
#5103=VECTOR('',#17562,1.);
#5104=VECTOR('',#17563,1.);
#5105=VECTOR('',#17566,1.);
#5106=VECTOR('',#17567,1.);
#5107=VECTOR('',#17568,1.);
#5108=VECTOR('',#17571,1.);
#5109=VECTOR('',#17572,1.);
#5110=VECTOR('',#17573,1.);
#5111=VECTOR('',#17576,1.);
#5112=VECTOR('',#17577,1.);
#5113=VECTOR('',#17578,1.);
#5114=VECTOR('',#17581,1.);
#5115=VECTOR('',#17582,1.);
#5116=VECTOR('',#17583,1.);
#5117=VECTOR('',#17586,1.);
#5118=VECTOR('',#17587,1.);
#5119=VECTOR('',#17588,1.);
#5120=VECTOR('',#17591,1.);
#5121=VECTOR('',#17592,1.);
#5122=VECTOR('',#17593,1.);
#5123=VECTOR('',#17596,1.);
#5124=VECTOR('',#17597,1.);
#5125=VECTOR('',#17598,1.);
#5126=VECTOR('',#17601,1.);
#5127=VECTOR('',#17602,1.);
#5128=VECTOR('',#17603,1.);
#5129=VECTOR('',#17606,1.);
#5130=VECTOR('',#17607,1.);
#5131=VECTOR('',#17608,1.);
#5132=VECTOR('',#17611,1.);
#5133=VECTOR('',#17612,1.);
#5134=VECTOR('',#17613,1.);
#5135=VECTOR('',#17616,1.);
#5136=VECTOR('',#17617,1.);
#5137=VECTOR('',#17618,1.);
#5138=VECTOR('',#17621,1.);
#5139=VECTOR('',#17622,1.);
#5140=VECTOR('',#17623,1.);
#5141=VECTOR('',#17626,1.);
#5142=VECTOR('',#17627,1.);
#5143=VECTOR('',#17628,1.);
#5144=VECTOR('',#17631,1.);
#5145=VECTOR('',#17632,1.);
#5146=VECTOR('',#17633,1.);
#5147=VECTOR('',#17636,1.);
#5148=VECTOR('',#17637,1.);
#5149=VECTOR('',#17638,1.);
#5150=VECTOR('',#17641,1.);
#5151=VECTOR('',#17642,1.);
#5152=VECTOR('',#17643,1.);
#5153=VECTOR('',#17646,1.);
#5154=VECTOR('',#17647,1.);
#5155=VECTOR('',#17648,1.);
#5156=VECTOR('',#17651,1.);
#5157=VECTOR('',#17652,1.);
#5158=VECTOR('',#17653,1.);
#5159=VECTOR('',#17656,1.);
#5160=VECTOR('',#17657,1.);
#5161=VECTOR('',#17658,1.);
#5162=VECTOR('',#17661,1.);
#5163=VECTOR('',#17662,1.);
#5164=VECTOR('',#17663,1.);
#5165=VECTOR('',#17666,1.);
#5166=VECTOR('',#17667,1.);
#5167=VECTOR('',#17668,1.);
#5168=VECTOR('',#17671,1.);
#5169=VECTOR('',#17672,1.);
#5170=VECTOR('',#17673,1.);
#5171=VECTOR('',#17676,1.);
#5172=VECTOR('',#17677,1.);
#5173=VECTOR('',#17678,1.);
#5174=VECTOR('',#17681,1.);
#5175=VECTOR('',#17682,1.);
#5176=VECTOR('',#17683,1.);
#5177=VECTOR('',#17686,1.);
#5178=VECTOR('',#17687,1.);
#5179=VECTOR('',#17688,1.);
#5180=VECTOR('',#17691,1.);
#5181=VECTOR('',#17692,1.);
#5182=VECTOR('',#17693,1.);
#5183=VECTOR('',#17696,1.);
#5184=VECTOR('',#17697,1.);
#5185=VECTOR('',#17698,1.);
#5186=VECTOR('',#17701,1.);
#5187=VECTOR('',#17702,1.);
#5188=VECTOR('',#17703,1.);
#5189=VECTOR('',#17706,1.);
#5190=VECTOR('',#17707,1.);
#5191=VECTOR('',#17708,1.);
#5192=VECTOR('',#17711,1.);
#5193=VECTOR('',#17712,1.);
#5194=VECTOR('',#17713,1.);
#5195=VECTOR('',#17716,1.);
#5196=VECTOR('',#17717,1.);
#5197=VECTOR('',#17718,1.);
#5198=VECTOR('',#17721,1.);
#5199=VECTOR('',#17722,1.);
#5200=VECTOR('',#17723,1.);
#5201=VECTOR('',#17726,1.);
#5202=VECTOR('',#17727,1.);
#5203=VECTOR('',#17728,1.);
#5204=VECTOR('',#17731,1.);
#5205=VECTOR('',#17732,1.);
#5206=VECTOR('',#17733,1.);
#5207=VECTOR('',#17736,1.);
#5208=VECTOR('',#17737,1.);
#5209=VECTOR('',#17738,1.);
#5210=VECTOR('',#17741,1.);
#5211=VECTOR('',#17742,1.);
#5212=VECTOR('',#17743,1.);
#5213=VECTOR('',#17746,1.);
#5214=VECTOR('',#17747,1.);
#5215=VECTOR('',#17748,1.);
#5216=VECTOR('',#17751,1.);
#5217=VECTOR('',#17752,1.);
#5218=VECTOR('',#17753,1.);
#5219=VECTOR('',#17756,1.);
#5220=VECTOR('',#17757,1.);
#5221=VECTOR('',#17758,1.);
#5222=VECTOR('',#17761,1.);
#5223=VECTOR('',#17762,1.);
#5224=VECTOR('',#17763,1.);
#5225=VECTOR('',#17766,1.);
#5226=VECTOR('',#17767,1.);
#5227=VECTOR('',#17768,1.);
#5228=VECTOR('',#17771,1.);
#5229=VECTOR('',#17772,1.);
#5230=VECTOR('',#17773,1.);
#5231=VECTOR('',#17776,1.);
#5232=VECTOR('',#17777,1.);
#5233=VECTOR('',#17778,1.);
#5234=VECTOR('',#17781,1.);
#5235=VECTOR('',#17782,1.);
#5236=VECTOR('',#17783,1.);
#5237=VECTOR('',#17786,1.);
#5238=VECTOR('',#17787,1.);
#5239=VECTOR('',#17788,1.);
#5240=VECTOR('',#17791,1.);
#5241=VECTOR('',#17792,1.);
#5242=VECTOR('',#17793,1.);
#5243=VECTOR('',#17796,1.);
#5244=VECTOR('',#17797,1.);
#5245=VECTOR('',#17798,1.);
#5246=VECTOR('',#17801,1.);
#5247=VECTOR('',#17802,1.);
#5248=VECTOR('',#17803,1.);
#5249=VECTOR('',#17806,1.);
#5250=VECTOR('',#17807,1.);
#5251=VECTOR('',#17808,1.);
#5252=VECTOR('',#17811,1.);
#5253=VECTOR('',#17812,1.);
#5254=VECTOR('',#17813,1.);
#5255=VECTOR('',#17816,1.);
#5256=VECTOR('',#17817,1.);
#5257=VECTOR('',#17818,1.);
#5258=VECTOR('',#17821,1.);
#5259=VECTOR('',#17822,1.);
#5260=VECTOR('',#17823,1.);
#5261=VECTOR('',#17826,1.);
#5262=VECTOR('',#17827,1.);
#5263=VECTOR('',#17828,1.);
#5264=VECTOR('',#17831,1.);
#5265=VECTOR('',#17832,1.);
#5266=VECTOR('',#17833,1.);
#5267=VECTOR('',#17836,1.);
#5268=VECTOR('',#17837,1.);
#5269=VECTOR('',#17838,1.);
#5270=VECTOR('',#17841,1.);
#5271=VECTOR('',#17842,1.);
#5272=VECTOR('',#17843,1.);
#5273=VECTOR('',#17846,1.);
#5274=VECTOR('',#17847,1.);
#5275=VECTOR('',#17848,1.);
#5276=VECTOR('',#17851,1.);
#5277=VECTOR('',#17852,1.);
#5278=VECTOR('',#17853,1.);
#5279=VECTOR('',#17856,1.);
#5280=VECTOR('',#17857,1.);
#5281=VECTOR('',#17858,1.);
#5282=VECTOR('',#17861,1.);
#5283=VECTOR('',#17862,1.);
#5284=VECTOR('',#17863,1.);
#5285=VECTOR('',#17866,1.);
#5286=VECTOR('',#17867,1.);
#5287=VECTOR('',#17868,1.);
#5288=VECTOR('',#17871,1.);
#5289=VECTOR('',#17872,1.);
#5290=VECTOR('',#17873,1.);
#5291=VECTOR('',#17876,1.);
#5292=VECTOR('',#17877,1.);
#5293=VECTOR('',#17878,1.);
#5294=VECTOR('',#17881,1.);
#5295=VECTOR('',#17882,1.);
#5296=VECTOR('',#17883,1.);
#5297=VECTOR('',#17886,1.);
#5298=VECTOR('',#17887,1.);
#5299=VECTOR('',#17888,1.);
#5300=VECTOR('',#17891,1.);
#5301=VECTOR('',#17892,1.);
#5302=VECTOR('',#17893,1.);
#5303=VECTOR('',#17896,1.);
#5304=VECTOR('',#17897,1.);
#5305=VECTOR('',#17898,1.);
#5306=VECTOR('',#17901,1.);
#5307=VECTOR('',#17902,1.);
#5308=VECTOR('',#17903,1.);
#5309=VECTOR('',#17906,1.);
#5310=VECTOR('',#17907,1.);
#5311=VECTOR('',#17908,1.);
#5312=VECTOR('',#17911,1.);
#5313=VECTOR('',#17912,1.);
#5314=VECTOR('',#17913,1.);
#5315=VECTOR('',#17916,1.);
#5316=VECTOR('',#17917,1.);
#5317=VECTOR('',#17918,1.);
#5318=VECTOR('',#17921,1.);
#5319=VECTOR('',#17922,1.);
#5320=VECTOR('',#17923,1.);
#5321=VECTOR('',#17926,1.);
#5322=VECTOR('',#17927,1.);
#5323=VECTOR('',#17928,1.);
#5324=VECTOR('',#17931,1.);
#5325=VECTOR('',#17932,1.);
#5326=VECTOR('',#17933,1.);
#5327=VECTOR('',#17936,1.);
#5328=VECTOR('',#17937,1.);
#5329=VECTOR('',#17938,1.);
#5330=VECTOR('',#17941,1.);
#5331=VECTOR('',#17942,1.);
#5332=VECTOR('',#17943,1.);
#5333=VECTOR('',#17946,1.);
#5334=VECTOR('',#17947,1.);
#5335=VECTOR('',#17948,1.);
#5336=VECTOR('',#17951,1.);
#5337=VECTOR('',#17952,1.);
#5338=VECTOR('',#17953,1.);
#5339=VECTOR('',#17956,1.);
#5340=VECTOR('',#17957,1.);
#5341=VECTOR('',#17958,1.);
#5342=VECTOR('',#17961,1.);
#5343=VECTOR('',#17962,1.);
#5344=VECTOR('',#17963,1.);
#5345=VECTOR('',#17966,1.);
#5346=VECTOR('',#17967,1.);
#5347=VECTOR('',#17968,1.);
#5348=VECTOR('',#17971,1.);
#5349=VECTOR('',#17972,1.);
#5350=VECTOR('',#17973,1.);
#5351=VECTOR('',#17976,1.);
#5352=VECTOR('',#17977,1.);
#5353=VECTOR('',#17978,1.);
#5354=VECTOR('',#17981,1.);
#5355=VECTOR('',#17982,1.);
#5356=VECTOR('',#17983,1.);
#5357=VECTOR('',#17986,1.);
#5358=VECTOR('',#17987,1.);
#5359=VECTOR('',#17988,1.);
#5360=VECTOR('',#17991,1.);
#5361=VECTOR('',#17992,1.);
#5362=VECTOR('',#17993,1.);
#5363=VECTOR('',#17996,1.);
#5364=VECTOR('',#17997,1.);
#5365=VECTOR('',#17998,1.);
#5366=VECTOR('',#18001,1.);
#5367=VECTOR('',#18002,1.);
#5368=VECTOR('',#18003,1.);
#5369=VECTOR('',#18006,1.);
#5370=VECTOR('',#18007,1.);
#5371=VECTOR('',#18008,1.);
#5372=VECTOR('',#18011,1.);
#5373=VECTOR('',#18012,1.);
#5374=VECTOR('',#18013,1.);
#5375=VECTOR('',#18016,1.);
#5376=VECTOR('',#18017,1.);
#5377=VECTOR('',#18018,1.);
#5378=VECTOR('',#18021,1.);
#5379=VECTOR('',#18022,1.);
#5380=VECTOR('',#18023,1.);
#5381=VECTOR('',#18026,1.);
#5382=VECTOR('',#18027,1.);
#5383=VECTOR('',#18028,1.);
#5384=VECTOR('',#18031,1.);
#5385=VECTOR('',#18032,1.);
#5386=VECTOR('',#18033,1.);
#5387=VECTOR('',#18036,1.);
#5388=VECTOR('',#18037,1.);
#5389=VECTOR('',#18038,1.);
#5390=VECTOR('',#18041,1.);
#5391=VECTOR('',#18042,1.);
#5392=VECTOR('',#18043,1.);
#5393=VECTOR('',#18046,1.);
#5394=VECTOR('',#18047,1.);
#5395=VECTOR('',#18048,1.);
#5396=VECTOR('',#18051,1.);
#5397=VECTOR('',#18052,1.);
#5398=VECTOR('',#18053,1.);
#5399=VECTOR('',#18056,1.);
#5400=VECTOR('',#18057,1.);
#5401=VECTOR('',#18058,1.);
#5402=VECTOR('',#18061,1.);
#5403=VECTOR('',#18062,1.);
#5404=VECTOR('',#18063,1.);
#5405=VECTOR('',#18066,1.);
#5406=VECTOR('',#18067,1.);
#5407=VECTOR('',#18068,1.);
#5408=VECTOR('',#18071,1.);
#5409=VECTOR('',#18072,1.);
#5410=VECTOR('',#18073,1.);
#5411=VECTOR('',#18076,1.);
#5412=VECTOR('',#18077,1.);
#6073=CIRCLE('',#14964,0.164999999999999);
#6074=CIRCLE('',#14965,0.164999999999999);
#6075=CIRCLE('',#14968,0.165);
#6076=CIRCLE('',#14969,0.165);
#6077=CIRCLE('',#14972,0.165);
#6078=CIRCLE('',#14973,0.165);
#6079=CIRCLE('',#14976,0.164999999999999);
#6080=CIRCLE('',#14977,0.164999999999999);
#6758=VERTEX_POINT('',#21456);
#6759=VERTEX_POINT('',#21458);
#6760=VERTEX_POINT('',#21463);
#6761=VERTEX_POINT('',#21465);
#6762=VERTEX_POINT('',#21470);
#6763=VERTEX_POINT('',#21472);
#6764=VERTEX_POINT('',#21477);
#6765=VERTEX_POINT('',#21479);
#6766=VERTEX_POINT('',#21484);
#6767=VERTEX_POINT('',#21485);
#6768=VERTEX_POINT('',#21487);
#6769=VERTEX_POINT('',#21489);
#6770=VERTEX_POINT('',#21493);
#6771=VERTEX_POINT('',#21495);
#6772=VERTEX_POINT('',#21499);
#6773=VERTEX_POINT('',#21501);
#6774=VERTEX_POINT('',#21505);
#6775=VERTEX_POINT('',#21507);
#6776=VERTEX_POINT('',#21511);
#6777=VERTEX_POINT('',#21513);
#6778=VERTEX_POINT('',#21517);
#6779=VERTEX_POINT('',#21519);
#6780=VERTEX_POINT('',#21523);
#6781=VERTEX_POINT('',#21525);
#6782=VERTEX_POINT('',#21529);
#6783=VERTEX_POINT('',#21531);
#6784=VERTEX_POINT('',#21535);
#6785=VERTEX_POINT('',#21537);
#6786=VERTEX_POINT('',#21541);
#6787=VERTEX_POINT('',#21543);
#6788=VERTEX_POINT('',#21547);
#6789=VERTEX_POINT('',#21549);
#6790=VERTEX_POINT('',#21553);
#6791=VERTEX_POINT('',#21555);
#6792=VERTEX_POINT('',#21559);
#6793=VERTEX_POINT('',#21561);
#6794=VERTEX_POINT('',#21565);
#6795=VERTEX_POINT('',#21567);
#6796=VERTEX_POINT('',#21571);
#6797=VERTEX_POINT('',#21573);
#6798=VERTEX_POINT('',#21577);
#6799=VERTEX_POINT('',#21579);
#6800=VERTEX_POINT('',#21583);
#6801=VERTEX_POINT('',#21585);
#6802=VERTEX_POINT('',#21589);
#6803=VERTEX_POINT('',#21591);
#6804=VERTEX_POINT('',#21595);
#6805=VERTEX_POINT('',#21597);
#6806=VERTEX_POINT('',#21601);
#6807=VERTEX_POINT('',#21603);
#6808=VERTEX_POINT('',#21607);
#6809=VERTEX_POINT('',#21609);
#6810=VERTEX_POINT('',#21613);
#6811=VERTEX_POINT('',#21615);
#6812=VERTEX_POINT('',#21619);
#6813=VERTEX_POINT('',#21621);
#6814=VERTEX_POINT('',#21625);
#6815=VERTEX_POINT('',#21627);
#6816=VERTEX_POINT('',#21631);
#6817=VERTEX_POINT('',#21633);
#6818=VERTEX_POINT('',#21637);
#6819=VERTEX_POINT('',#21639);
#6820=VERTEX_POINT('',#21643);
#6821=VERTEX_POINT('',#21645);
#6822=VERTEX_POINT('',#21649);
#6823=VERTEX_POINT('',#21651);
#6824=VERTEX_POINT('',#21655);
#6825=VERTEX_POINT('',#21657);
#6826=VERTEX_POINT('',#21661);
#6827=VERTEX_POINT('',#21663);
#6828=VERTEX_POINT('',#21667);
#6829=VERTEX_POINT('',#21669);
#6830=VERTEX_POINT('',#21673);
#6831=VERTEX_POINT('',#21675);
#6832=VERTEX_POINT('',#21679);
#6833=VERTEX_POINT('',#21681);
#6834=VERTEX_POINT('',#21685);
#6835=VERTEX_POINT('',#21687);
#6836=VERTEX_POINT('',#21691);
#6837=VERTEX_POINT('',#21693);
#6838=VERTEX_POINT('',#21697);
#6839=VERTEX_POINT('',#21699);
#6840=VERTEX_POINT('',#21703);
#6841=VERTEX_POINT('',#21705);
#6842=VERTEX_POINT('',#21709);
#6843=VERTEX_POINT('',#21711);
#6844=VERTEX_POINT('',#21715);
#6845=VERTEX_POINT('',#21717);
#6846=VERTEX_POINT('',#21721);
#6847=VERTEX_POINT('',#21723);
#6848=VERTEX_POINT('',#21727);
#6849=VERTEX_POINT('',#21729);
#6850=VERTEX_POINT('',#21733);
#6851=VERTEX_POINT('',#21735);
#6852=VERTEX_POINT('',#21739);
#6853=VERTEX_POINT('',#21741);
#6854=VERTEX_POINT('',#21745);
#6855=VERTEX_POINT('',#21747);
#6856=VERTEX_POINT('',#21751);
#6857=VERTEX_POINT('',#21753);
#6858=VERTEX_POINT('',#21757);
#6859=VERTEX_POINT('',#21759);
#6860=VERTEX_POINT('',#21763);
#6861=VERTEX_POINT('',#21765);
#6862=VERTEX_POINT('',#21769);
#6863=VERTEX_POINT('',#21771);
#6864=VERTEX_POINT('',#21775);
#6865=VERTEX_POINT('',#21777);
#6866=VERTEX_POINT('',#21781);
#6867=VERTEX_POINT('',#21783);
#6868=VERTEX_POINT('',#21787);
#6869=VERTEX_POINT('',#21789);
#6870=VERTEX_POINT('',#21793);
#6871=VERTEX_POINT('',#21795);
#6872=VERTEX_POINT('',#21799);
#6873=VERTEX_POINT('',#21801);
#6874=VERTEX_POINT('',#21805);
#6875=VERTEX_POINT('',#21807);
#6876=VERTEX_POINT('',#21811);
#6877=VERTEX_POINT('',#21813);
#6878=VERTEX_POINT('',#21817);
#6879=VERTEX_POINT('',#21819);
#6880=VERTEX_POINT('',#21823);
#6881=VERTEX_POINT('',#21825);
#6882=VERTEX_POINT('',#21829);
#6883=VERTEX_POINT('',#21831);
#6884=VERTEX_POINT('',#21835);
#6885=VERTEX_POINT('',#21837);
#6886=VERTEX_POINT('',#21841);
#6887=VERTEX_POINT('',#21843);
#6888=VERTEX_POINT('',#21847);
#6889=VERTEX_POINT('',#21849);
#6890=VERTEX_POINT('',#21853);
#6891=VERTEX_POINT('',#21855);
#6892=VERTEX_POINT('',#21859);
#6893=VERTEX_POINT('',#21861);
#6894=VERTEX_POINT('',#21865);
#6895=VERTEX_POINT('',#21867);
#6896=VERTEX_POINT('',#21871);
#6897=VERTEX_POINT('',#21873);
#6898=VERTEX_POINT('',#21877);
#6899=VERTEX_POINT('',#21879);
#6900=VERTEX_POINT('',#21883);
#6901=VERTEX_POINT('',#21885);
#6902=VERTEX_POINT('',#21889);
#6903=VERTEX_POINT('',#21891);
#6904=VERTEX_POINT('',#21895);
#6905=VERTEX_POINT('',#21897);
#6906=VERTEX_POINT('',#21901);
#6907=VERTEX_POINT('',#21903);
#6908=VERTEX_POINT('',#21907);
#6909=VERTEX_POINT('',#21909);
#6910=VERTEX_POINT('',#21913);
#6911=VERTEX_POINT('',#21915);
#6912=VERTEX_POINT('',#21919);
#6913=VERTEX_POINT('',#21921);
#6914=VERTEX_POINT('',#21925);
#6915=VERTEX_POINT('',#21927);
#6916=VERTEX_POINT('',#21931);
#6917=VERTEX_POINT('',#21933);
#6918=VERTEX_POINT('',#21937);
#6919=VERTEX_POINT('',#21939);
#6920=VERTEX_POINT('',#21943);
#6921=VERTEX_POINT('',#21945);
#6922=VERTEX_POINT('',#21949);
#6923=VERTEX_POINT('',#21951);
#6924=VERTEX_POINT('',#21955);
#6925=VERTEX_POINT('',#21957);
#6926=VERTEX_POINT('',#21961);
#6927=VERTEX_POINT('',#21963);
#6928=VERTEX_POINT('',#21967);
#6929=VERTEX_POINT('',#21969);
#6930=VERTEX_POINT('',#21973);
#6931=VERTEX_POINT('',#21975);
#6932=VERTEX_POINT('',#21979);
#6933=VERTEX_POINT('',#21981);
#6934=VERTEX_POINT('',#21985);
#6935=VERTEX_POINT('',#21987);
#6936=VERTEX_POINT('',#21991);
#6937=VERTEX_POINT('',#21993);
#6938=VERTEX_POINT('',#21997);
#6939=VERTEX_POINT('',#21999);
#6940=VERTEX_POINT('',#22003);
#6941=VERTEX_POINT('',#22005);
#6942=VERTEX_POINT('',#22009);
#6943=VERTEX_POINT('',#22011);
#6944=VERTEX_POINT('',#22015);
#6945=VERTEX_POINT('',#22017);
#6946=VERTEX_POINT('',#22021);
#6947=VERTEX_POINT('',#22023);
#6948=VERTEX_POINT('',#22027);
#6949=VERTEX_POINT('',#22029);
#6950=VERTEX_POINT('',#22033);
#6951=VERTEX_POINT('',#22035);
#6952=VERTEX_POINT('',#22039);
#6953=VERTEX_POINT('',#22041);
#6954=VERTEX_POINT('',#22045);
#6955=VERTEX_POINT('',#22047);
#6956=VERTEX_POINT('',#22051);
#6957=VERTEX_POINT('',#22053);
#6958=VERTEX_POINT('',#22057);
#6959=VERTEX_POINT('',#22059);
#6960=VERTEX_POINT('',#22063);
#6961=VERTEX_POINT('',#22065);
#6962=VERTEX_POINT('',#22069);
#6963=VERTEX_POINT('',#22071);
#6964=VERTEX_POINT('',#22075);
#6965=VERTEX_POINT('',#22077);
#6966=VERTEX_POINT('',#22081);
#6967=VERTEX_POINT('',#22083);
#6968=VERTEX_POINT('',#22087);
#6969=VERTEX_POINT('',#22089);
#6970=VERTEX_POINT('',#22093);
#6971=VERTEX_POINT('',#22095);
#6972=VERTEX_POINT('',#22099);
#6973=VERTEX_POINT('',#22101);
#6974=VERTEX_POINT('',#22105);
#6975=VERTEX_POINT('',#22107);
#6976=VERTEX_POINT('',#22111);
#6977=VERTEX_POINT('',#22113);
#6978=VERTEX_POINT('',#22117);
#6979=VERTEX_POINT('',#22119);
#6980=VERTEX_POINT('',#22123);
#6981=VERTEX_POINT('',#22125);
#6982=VERTEX_POINT('',#22129);
#6983=VERTEX_POINT('',#22131);
#6984=VERTEX_POINT('',#22135);
#6985=VERTEX_POINT('',#22137);
#6986=VERTEX_POINT('',#22141);
#6987=VERTEX_POINT('',#22143);
#6988=VERTEX_POINT('',#22147);
#6989=VERTEX_POINT('',#22149);
#6990=VERTEX_POINT('',#22153);
#6991=VERTEX_POINT('',#22155);
#6992=VERTEX_POINT('',#22159);
#6993=VERTEX_POINT('',#22161);
#6994=VERTEX_POINT('',#22165);
#6995=VERTEX_POINT('',#22167);
#6996=VERTEX_POINT('',#22171);
#6997=VERTEX_POINT('',#22173);
#6998=VERTEX_POINT('',#22177);
#6999=VERTEX_POINT('',#22179);
#7000=VERTEX_POINT('',#22183);
#7001=VERTEX_POINT('',#22185);
#7002=VERTEX_POINT('',#22189);
#7003=VERTEX_POINT('',#22191);
#7004=VERTEX_POINT('',#22195);
#7005=VERTEX_POINT('',#22197);
#7006=VERTEX_POINT('',#22201);
#7007=VERTEX_POINT('',#22203);
#7008=VERTEX_POINT('',#22207);
#7009=VERTEX_POINT('',#22209);
#7010=VERTEX_POINT('',#22213);
#7011=VERTEX_POINT('',#22215);
#7012=VERTEX_POINT('',#22219);
#7013=VERTEX_POINT('',#22221);
#7014=VERTEX_POINT('',#22225);
#7015=VERTEX_POINT('',#22227);
#7016=VERTEX_POINT('',#22231);
#7017=VERTEX_POINT('',#22233);
#7018=VERTEX_POINT('',#22237);
#7019=VERTEX_POINT('',#22239);
#7020=VERTEX_POINT('',#22243);
#7021=VERTEX_POINT('',#22245);
#8222=EDGE_CURVE('',#6758,#6758,#6073,.T.);
#8223=EDGE_CURVE('',#6758,#6759,#3734,.T.);
#8224=EDGE_CURVE('',#6759,#6759,#6074,.T.);
#8225=EDGE_CURVE('',#6760,#6760,#6075,.T.);
#8226=EDGE_CURVE('',#6760,#6761,#3735,.T.);
#8227=EDGE_CURVE('',#6761,#6761,#6076,.T.);
#8228=EDGE_CURVE('',#6762,#6762,#6077,.T.);
#8229=EDGE_CURVE('',#6762,#6763,#3736,.T.);
#8230=EDGE_CURVE('',#6763,#6763,#6078,.T.);
#8231=EDGE_CURVE('',#6764,#6764,#6079,.T.);
#8232=EDGE_CURVE('',#6764,#6765,#3737,.T.);
#8233=EDGE_CURVE('',#6765,#6765,#6080,.T.);
#8234=EDGE_CURVE('',#6766,#6767,#3738,.T.);
#8235=EDGE_CURVE('',#6766,#6768,#3739,.T.);
#8236=EDGE_CURVE('',#6769,#6768,#3740,.T.);
#8237=EDGE_CURVE('',#6767,#6769,#3741,.T.);
#8238=EDGE_CURVE('',#6767,#6770,#3742,.T.);
#8239=EDGE_CURVE('',#6771,#6769,#3743,.T.);
#8240=EDGE_CURVE('',#6770,#6771,#3744,.T.);
#8241=EDGE_CURVE('',#6770,#6772,#3745,.T.);
#8242=EDGE_CURVE('',#6773,#6771,#3746,.T.);
#8243=EDGE_CURVE('',#6772,#6773,#3747,.T.);
#8244=EDGE_CURVE('',#6772,#6774,#3748,.T.);
#8245=EDGE_CURVE('',#6775,#6773,#3749,.T.);
#8246=EDGE_CURVE('',#6774,#6775,#3750,.T.);
#8247=EDGE_CURVE('',#6774,#6776,#3751,.T.);
#8248=EDGE_CURVE('',#6777,#6775,#3752,.T.);
#8249=EDGE_CURVE('',#6776,#6777,#3753,.T.);
#8250=EDGE_CURVE('',#6776,#6778,#3754,.T.);
#8251=EDGE_CURVE('',#6779,#6777,#3755,.T.);
#8252=EDGE_CURVE('',#6778,#6779,#3756,.T.);
#8253=EDGE_CURVE('',#6778,#6780,#3757,.T.);
#8254=EDGE_CURVE('',#6781,#6779,#3758,.T.);
#8255=EDGE_CURVE('',#6780,#6781,#3759,.T.);
#8256=EDGE_CURVE('',#6780,#6782,#3760,.T.);
#8257=EDGE_CURVE('',#6783,#6781,#3761,.T.);
#8258=EDGE_CURVE('',#6782,#6783,#3762,.T.);
#8259=EDGE_CURVE('',#6782,#6784,#3763,.T.);
#8260=EDGE_CURVE('',#6785,#6783,#3764,.T.);
#8261=EDGE_CURVE('',#6784,#6785,#3765,.T.);
#8262=EDGE_CURVE('',#6784,#6786,#3766,.T.);
#8263=EDGE_CURVE('',#6787,#6785,#3767,.T.);
#8264=EDGE_CURVE('',#6786,#6787,#3768,.T.);
#8265=EDGE_CURVE('',#6786,#6788,#3769,.T.);
#8266=EDGE_CURVE('',#6789,#6787,#3770,.T.);
#8267=EDGE_CURVE('',#6788,#6789,#3771,.T.);
#8268=EDGE_CURVE('',#6788,#6790,#3772,.T.);
#8269=EDGE_CURVE('',#6791,#6789,#3773,.T.);
#8270=EDGE_CURVE('',#6790,#6791,#3774,.T.);
#8271=EDGE_CURVE('',#6790,#6792,#3775,.T.);
#8272=EDGE_CURVE('',#6793,#6791,#3776,.T.);
#8273=EDGE_CURVE('',#6792,#6793,#3777,.T.);
#8274=EDGE_CURVE('',#6792,#6794,#3778,.T.);
#8275=EDGE_CURVE('',#6795,#6793,#3779,.T.);
#8276=EDGE_CURVE('',#6794,#6795,#3780,.T.);
#8277=EDGE_CURVE('',#6794,#6796,#3781,.T.);
#8278=EDGE_CURVE('',#6797,#6795,#3782,.T.);
#8279=EDGE_CURVE('',#6796,#6797,#3783,.T.);
#8280=EDGE_CURVE('',#6796,#6798,#3784,.T.);
#8281=EDGE_CURVE('',#6799,#6797,#3785,.T.);
#8282=EDGE_CURVE('',#6798,#6799,#3786,.T.);
#8283=EDGE_CURVE('',#6798,#6800,#3787,.T.);
#8284=EDGE_CURVE('',#6801,#6799,#3788,.T.);
#8285=EDGE_CURVE('',#6800,#6801,#3789,.T.);
#8286=EDGE_CURVE('',#6800,#6802,#3790,.T.);
#8287=EDGE_CURVE('',#6803,#6801,#3791,.T.);
#8288=EDGE_CURVE('',#6802,#6803,#3792,.T.);
#8289=EDGE_CURVE('',#6802,#6804,#3793,.T.);
#8290=EDGE_CURVE('',#6805,#6803,#3794,.T.);
#8291=EDGE_CURVE('',#6804,#6805,#3795,.T.);
#8292=EDGE_CURVE('',#6804,#6806,#3796,.T.);
#8293=EDGE_CURVE('',#6807,#6805,#3797,.T.);
#8294=EDGE_CURVE('',#6806,#6807,#3798,.T.);
#8295=EDGE_CURVE('',#6806,#6808,#3799,.T.);
#8296=EDGE_CURVE('',#6809,#6807,#3800,.T.);
#8297=EDGE_CURVE('',#6808,#6809,#3801,.T.);
#8298=EDGE_CURVE('',#6808,#6810,#3802,.T.);
#8299=EDGE_CURVE('',#6811,#6809,#3803,.T.);
#8300=EDGE_CURVE('',#6810,#6811,#3804,.T.);
#8301=EDGE_CURVE('',#6810,#6812,#3805,.T.);
#8302=EDGE_CURVE('',#6813,#6811,#3806,.T.);
#8303=EDGE_CURVE('',#6812,#6813,#3807,.T.);
#8304=EDGE_CURVE('',#6812,#6814,#3808,.T.);
#8305=EDGE_CURVE('',#6815,#6813,#3809,.T.);
#8306=EDGE_CURVE('',#6814,#6815,#3810,.T.);
#8307=EDGE_CURVE('',#6814,#6816,#3811,.T.);
#8308=EDGE_CURVE('',#6817,#6815,#3812,.T.);
#8309=EDGE_CURVE('',#6816,#6817,#3813,.T.);
#8310=EDGE_CURVE('',#6816,#6818,#3814,.T.);
#8311=EDGE_CURVE('',#6819,#6817,#3815,.T.);
#8312=EDGE_CURVE('',#6818,#6819,#3816,.T.);
#8313=EDGE_CURVE('',#6818,#6820,#3817,.T.);
#8314=EDGE_CURVE('',#6821,#6819,#3818,.T.);
#8315=EDGE_CURVE('',#6820,#6821,#3819,.T.);
#8316=EDGE_CURVE('',#6820,#6822,#3820,.T.);
#8317=EDGE_CURVE('',#6823,#6821,#3821,.T.);
#8318=EDGE_CURVE('',#6822,#6823,#3822,.T.);
#8319=EDGE_CURVE('',#6822,#6824,#3823,.T.);
#8320=EDGE_CURVE('',#6825,#6823,#3824,.T.);
#8321=EDGE_CURVE('',#6824,#6825,#3825,.T.);
#8322=EDGE_CURVE('',#6824,#6826,#3826,.T.);
#8323=EDGE_CURVE('',#6827,#6825,#3827,.T.);
#8324=EDGE_CURVE('',#6826,#6827,#3828,.T.);
#8325=EDGE_CURVE('',#6826,#6828,#3829,.T.);
#8326=EDGE_CURVE('',#6829,#6827,#3830,.T.);
#8327=EDGE_CURVE('',#6828,#6829,#3831,.T.);
#8328=EDGE_CURVE('',#6828,#6830,#3832,.T.);
#8329=EDGE_CURVE('',#6831,#6829,#3833,.T.);
#8330=EDGE_CURVE('',#6830,#6831,#3834,.T.);
#8331=EDGE_CURVE('',#6830,#6832,#3835,.T.);
#8332=EDGE_CURVE('',#6833,#6831,#3836,.T.);
#8333=EDGE_CURVE('',#6832,#6833,#3837,.T.);
#8334=EDGE_CURVE('',#6832,#6834,#3838,.T.);
#8335=EDGE_CURVE('',#6835,#6833,#3839,.T.);
#8336=EDGE_CURVE('',#6834,#6835,#3840,.T.);
#8337=EDGE_CURVE('',#6834,#6836,#3841,.T.);
#8338=EDGE_CURVE('',#6837,#6835,#3842,.T.);
#8339=EDGE_CURVE('',#6836,#6837,#3843,.T.);
#8340=EDGE_CURVE('',#6836,#6838,#3844,.T.);
#8341=EDGE_CURVE('',#6839,#6837,#3845,.T.);
#8342=EDGE_CURVE('',#6838,#6839,#3846,.T.);
#8343=EDGE_CURVE('',#6838,#6840,#3847,.T.);
#8344=EDGE_CURVE('',#6841,#6839,#3848,.T.);
#8345=EDGE_CURVE('',#6840,#6841,#3849,.T.);
#8346=EDGE_CURVE('',#6840,#6842,#3850,.T.);
#8347=EDGE_CURVE('',#6843,#6841,#3851,.T.);
#8348=EDGE_CURVE('',#6842,#6843,#3852,.T.);
#8349=EDGE_CURVE('',#6842,#6844,#3853,.T.);
#8350=EDGE_CURVE('',#6845,#6843,#3854,.T.);
#8351=EDGE_CURVE('',#6844,#6845,#3855,.T.);
#8352=EDGE_CURVE('',#6844,#6846,#3856,.T.);
#8353=EDGE_CURVE('',#6847,#6845,#3857,.T.);
#8354=EDGE_CURVE('',#6846,#6847,#3858,.T.);
#8355=EDGE_CURVE('',#6846,#6848,#3859,.T.);
#8356=EDGE_CURVE('',#6849,#6847,#3860,.T.);
#8357=EDGE_CURVE('',#6848,#6849,#3861,.T.);
#8358=EDGE_CURVE('',#6848,#6850,#3862,.T.);
#8359=EDGE_CURVE('',#6851,#6849,#3863,.T.);
#8360=EDGE_CURVE('',#6850,#6851,#3864,.T.);
#8361=EDGE_CURVE('',#6850,#6852,#3865,.T.);
#8362=EDGE_CURVE('',#6853,#6851,#3866,.T.);
#8363=EDGE_CURVE('',#6852,#6853,#3867,.T.);
#8364=EDGE_CURVE('',#6852,#6854,#3868,.T.);
#8365=EDGE_CURVE('',#6855,#6853,#3869,.T.);
#8366=EDGE_CURVE('',#6854,#6855,#3870,.T.);
#8367=EDGE_CURVE('',#6854,#6856,#3871,.T.);
#8368=EDGE_CURVE('',#6857,#6855,#3872,.T.);
#8369=EDGE_CURVE('',#6856,#6857,#3873,.T.);
#8370=EDGE_CURVE('',#6856,#6858,#3874,.T.);
#8371=EDGE_CURVE('',#6859,#6857,#3875,.T.);
#8372=EDGE_CURVE('',#6858,#6859,#3876,.T.);
#8373=EDGE_CURVE('',#6858,#6860,#3877,.T.);
#8374=EDGE_CURVE('',#6861,#6859,#3878,.T.);
#8375=EDGE_CURVE('',#6860,#6861,#3879,.T.);
#8376=EDGE_CURVE('',#6860,#6862,#3880,.T.);
#8377=EDGE_CURVE('',#6863,#6861,#3881,.T.);
#8378=EDGE_CURVE('',#6862,#6863,#3882,.T.);
#8379=EDGE_CURVE('',#6862,#6864,#3883,.T.);
#8380=EDGE_CURVE('',#6865,#6863,#3884,.T.);
#8381=EDGE_CURVE('',#6864,#6865,#3885,.T.);
#8382=EDGE_CURVE('',#6864,#6866,#3886,.T.);
#8383=EDGE_CURVE('',#6867,#6865,#3887,.T.);
#8384=EDGE_CURVE('',#6866,#6867,#3888,.T.);
#8385=EDGE_CURVE('',#6866,#6868,#3889,.T.);
#8386=EDGE_CURVE('',#6869,#6867,#3890,.T.);
#8387=EDGE_CURVE('',#6868,#6869,#3891,.T.);
#8388=EDGE_CURVE('',#6868,#6870,#3892,.T.);
#8389=EDGE_CURVE('',#6871,#6869,#3893,.T.);
#8390=EDGE_CURVE('',#6870,#6871,#3894,.T.);
#8391=EDGE_CURVE('',#6870,#6872,#3895,.T.);
#8392=EDGE_CURVE('',#6873,#6871,#3896,.T.);
#8393=EDGE_CURVE('',#6872,#6873,#3897,.T.);
#8394=EDGE_CURVE('',#6872,#6874,#3898,.T.);
#8395=EDGE_CURVE('',#6875,#6873,#3899,.T.);
#8396=EDGE_CURVE('',#6874,#6875,#3900,.T.);
#8397=EDGE_CURVE('',#6874,#6876,#3901,.T.);
#8398=EDGE_CURVE('',#6877,#6875,#3902,.T.);
#8399=EDGE_CURVE('',#6876,#6877,#3903,.T.);
#8400=EDGE_CURVE('',#6876,#6878,#3904,.T.);
#8401=EDGE_CURVE('',#6879,#6877,#3905,.T.);
#8402=EDGE_CURVE('',#6878,#6879,#3906,.T.);
#8403=EDGE_CURVE('',#6878,#6880,#3907,.T.);
#8404=EDGE_CURVE('',#6881,#6879,#3908,.T.);
#8405=EDGE_CURVE('',#6880,#6881,#3909,.T.);
#8406=EDGE_CURVE('',#6880,#6882,#3910,.T.);
#8407=EDGE_CURVE('',#6883,#6881,#3911,.T.);
#8408=EDGE_CURVE('',#6882,#6883,#3912,.T.);
#8409=EDGE_CURVE('',#6882,#6884,#3913,.T.);
#8410=EDGE_CURVE('',#6885,#6883,#3914,.T.);
#8411=EDGE_CURVE('',#6884,#6885,#3915,.T.);
#8412=EDGE_CURVE('',#6884,#6886,#3916,.T.);
#8413=EDGE_CURVE('',#6887,#6885,#3917,.T.);
#8414=EDGE_CURVE('',#6886,#6887,#3918,.T.);
#8415=EDGE_CURVE('',#6886,#6888,#3919,.T.);
#8416=EDGE_CURVE('',#6889,#6887,#3920,.T.);
#8417=EDGE_CURVE('',#6888,#6889,#3921,.T.);
#8418=EDGE_CURVE('',#6888,#6890,#3922,.T.);
#8419=EDGE_CURVE('',#6891,#6889,#3923,.T.);
#8420=EDGE_CURVE('',#6890,#6891,#3924,.T.);
#8421=EDGE_CURVE('',#6890,#6892,#3925,.T.);
#8422=EDGE_CURVE('',#6893,#6891,#3926,.T.);
#8423=EDGE_CURVE('',#6892,#6893,#3927,.T.);
#8424=EDGE_CURVE('',#6892,#6894,#3928,.T.);
#8425=EDGE_CURVE('',#6895,#6893,#3929,.T.);
#8426=EDGE_CURVE('',#6894,#6895,#3930,.T.);
#8427=EDGE_CURVE('',#6894,#6896,#3931,.T.);
#8428=EDGE_CURVE('',#6897,#6895,#3932,.T.);
#8429=EDGE_CURVE('',#6896,#6897,#3933,.T.);
#8430=EDGE_CURVE('',#6896,#6898,#3934,.T.);
#8431=EDGE_CURVE('',#6899,#6897,#3935,.T.);
#8432=EDGE_CURVE('',#6898,#6899,#3936,.T.);
#8433=EDGE_CURVE('',#6898,#6900,#3937,.T.);
#8434=EDGE_CURVE('',#6901,#6899,#3938,.T.);
#8435=EDGE_CURVE('',#6900,#6901,#3939,.T.);
#8436=EDGE_CURVE('',#6900,#6902,#3940,.T.);
#8437=EDGE_CURVE('',#6903,#6901,#3941,.T.);
#8438=EDGE_CURVE('',#6902,#6903,#3942,.T.);
#8439=EDGE_CURVE('',#6902,#6904,#3943,.T.);
#8440=EDGE_CURVE('',#6905,#6903,#3944,.T.);
#8441=EDGE_CURVE('',#6904,#6905,#3945,.T.);
#8442=EDGE_CURVE('',#6904,#6906,#3946,.T.);
#8443=EDGE_CURVE('',#6907,#6905,#3947,.T.);
#8444=EDGE_CURVE('',#6906,#6907,#3948,.T.);
#8445=EDGE_CURVE('',#6906,#6908,#3949,.T.);
#8446=EDGE_CURVE('',#6909,#6907,#3950,.T.);
#8447=EDGE_CURVE('',#6908,#6909,#3951,.T.);
#8448=EDGE_CURVE('',#6908,#6910,#3952,.T.);
#8449=EDGE_CURVE('',#6911,#6909,#3953,.T.);
#8450=EDGE_CURVE('',#6910,#6911,#3954,.T.);
#8451=EDGE_CURVE('',#6910,#6912,#3955,.T.);
#8452=EDGE_CURVE('',#6913,#6911,#3956,.T.);
#8453=EDGE_CURVE('',#6912,#6913,#3957,.T.);
#8454=EDGE_CURVE('',#6912,#6914,#3958,.T.);
#8455=EDGE_CURVE('',#6915,#6913,#3959,.T.);
#8456=EDGE_CURVE('',#6914,#6915,#3960,.T.);
#8457=EDGE_CURVE('',#6914,#6916,#3961,.T.);
#8458=EDGE_CURVE('',#6917,#6915,#3962,.T.);
#8459=EDGE_CURVE('',#6916,#6917,#3963,.T.);
#8460=EDGE_CURVE('',#6916,#6918,#3964,.T.);
#8461=EDGE_CURVE('',#6919,#6917,#3965,.T.);
#8462=EDGE_CURVE('',#6918,#6919,#3966,.T.);
#8463=EDGE_CURVE('',#6918,#6920,#3967,.T.);
#8464=EDGE_CURVE('',#6921,#6919,#3968,.T.);
#8465=EDGE_CURVE('',#6920,#6921,#3969,.T.);
#8466=EDGE_CURVE('',#6920,#6922,#3970,.T.);
#8467=EDGE_CURVE('',#6923,#6921,#3971,.T.);
#8468=EDGE_CURVE('',#6922,#6923,#3972,.T.);
#8469=EDGE_CURVE('',#6922,#6924,#3973,.T.);
#8470=EDGE_CURVE('',#6925,#6923,#3974,.T.);
#8471=EDGE_CURVE('',#6924,#6925,#3975,.T.);
#8472=EDGE_CURVE('',#6924,#6926,#3976,.T.);
#8473=EDGE_CURVE('',#6927,#6925,#3977,.T.);
#8474=EDGE_CURVE('',#6926,#6927,#3978,.T.);
#8475=EDGE_CURVE('',#6926,#6928,#3979,.T.);
#8476=EDGE_CURVE('',#6929,#6927,#3980,.T.);
#8477=EDGE_CURVE('',#6928,#6929,#3981,.T.);
#8478=EDGE_CURVE('',#6928,#6930,#3982,.T.);
#8479=EDGE_CURVE('',#6931,#6929,#3983,.T.);
#8480=EDGE_CURVE('',#6930,#6931,#3984,.T.);
#8481=EDGE_CURVE('',#6930,#6932,#3985,.T.);
#8482=EDGE_CURVE('',#6933,#6931,#3986,.T.);
#8483=EDGE_CURVE('',#6932,#6933,#3987,.T.);
#8484=EDGE_CURVE('',#6932,#6934,#3988,.T.);
#8485=EDGE_CURVE('',#6935,#6933,#3989,.T.);
#8486=EDGE_CURVE('',#6934,#6935,#3990,.T.);
#8487=EDGE_CURVE('',#6934,#6936,#3991,.T.);
#8488=EDGE_CURVE('',#6937,#6935,#3992,.T.);
#8489=EDGE_CURVE('',#6936,#6937,#3993,.T.);
#8490=EDGE_CURVE('',#6936,#6938,#3994,.T.);
#8491=EDGE_CURVE('',#6939,#6937,#3995,.T.);
#8492=EDGE_CURVE('',#6938,#6939,#3996,.T.);
#8493=EDGE_CURVE('',#6938,#6940,#3997,.T.);
#8494=EDGE_CURVE('',#6941,#6939,#3998,.T.);
#8495=EDGE_CURVE('',#6940,#6941,#3999,.T.);
#8496=EDGE_CURVE('',#6940,#6942,#4000,.T.);
#8497=EDGE_CURVE('',#6943,#6941,#4001,.T.);
#8498=EDGE_CURVE('',#6942,#6943,#4002,.T.);
#8499=EDGE_CURVE('',#6942,#6944,#4003,.T.);
#8500=EDGE_CURVE('',#6945,#6943,#4004,.T.);
#8501=EDGE_CURVE('',#6944,#6945,#4005,.T.);
#8502=EDGE_CURVE('',#6944,#6946,#4006,.T.);
#8503=EDGE_CURVE('',#6947,#6945,#4007,.T.);
#8504=EDGE_CURVE('',#6946,#6947,#4008,.T.);
#8505=EDGE_CURVE('',#6946,#6948,#4009,.T.);
#8506=EDGE_CURVE('',#6949,#6947,#4010,.T.);
#8507=EDGE_CURVE('',#6948,#6949,#4011,.T.);
#8508=EDGE_CURVE('',#6948,#6950,#4012,.T.);
#8509=EDGE_CURVE('',#6951,#6949,#4013,.T.);
#8510=EDGE_CURVE('',#6950,#6951,#4014,.T.);
#8511=EDGE_CURVE('',#6950,#6952,#4015,.T.);
#8512=EDGE_CURVE('',#6953,#6951,#4016,.T.);
#8513=EDGE_CURVE('',#6952,#6953,#4017,.T.);
#8514=EDGE_CURVE('',#6952,#6954,#4018,.T.);
#8515=EDGE_CURVE('',#6955,#6953,#4019,.T.);
#8516=EDGE_CURVE('',#6954,#6955,#4020,.T.);
#8517=EDGE_CURVE('',#6954,#6956,#4021,.T.);
#8518=EDGE_CURVE('',#6957,#6955,#4022,.T.);
#8519=EDGE_CURVE('',#6956,#6957,#4023,.T.);
#8520=EDGE_CURVE('',#6956,#6958,#4024,.T.);
#8521=EDGE_CURVE('',#6959,#6957,#4025,.T.);
#8522=EDGE_CURVE('',#6958,#6959,#4026,.T.);
#8523=EDGE_CURVE('',#6958,#6960,#4027,.T.);
#8524=EDGE_CURVE('',#6961,#6959,#4028,.T.);
#8525=EDGE_CURVE('',#6960,#6961,#4029,.T.);
#8526=EDGE_CURVE('',#6960,#6962,#4030,.T.);
#8527=EDGE_CURVE('',#6963,#6961,#4031,.T.);
#8528=EDGE_CURVE('',#6962,#6963,#4032,.T.);
#8529=EDGE_CURVE('',#6962,#6964,#4033,.T.);
#8530=EDGE_CURVE('',#6965,#6963,#4034,.T.);
#8531=EDGE_CURVE('',#6964,#6965,#4035,.T.);
#8532=EDGE_CURVE('',#6964,#6966,#4036,.T.);
#8533=EDGE_CURVE('',#6967,#6965,#4037,.T.);
#8534=EDGE_CURVE('',#6966,#6967,#4038,.T.);
#8535=EDGE_CURVE('',#6966,#6968,#4039,.T.);
#8536=EDGE_CURVE('',#6969,#6967,#4040,.T.);
#8537=EDGE_CURVE('',#6968,#6969,#4041,.T.);
#8538=EDGE_CURVE('',#6968,#6970,#4042,.T.);
#8539=EDGE_CURVE('',#6971,#6969,#4043,.T.);
#8540=EDGE_CURVE('',#6970,#6971,#4044,.T.);
#8541=EDGE_CURVE('',#6970,#6972,#4045,.T.);
#8542=EDGE_CURVE('',#6973,#6971,#4046,.T.);
#8543=EDGE_CURVE('',#6972,#6973,#4047,.T.);
#8544=EDGE_CURVE('',#6972,#6974,#4048,.T.);
#8545=EDGE_CURVE('',#6975,#6973,#4049,.T.);
#8546=EDGE_CURVE('',#6974,#6975,#4050,.T.);
#8547=EDGE_CURVE('',#6974,#6976,#4051,.T.);
#8548=EDGE_CURVE('',#6977,#6975,#4052,.T.);
#8549=EDGE_CURVE('',#6976,#6977,#4053,.T.);
#8550=EDGE_CURVE('',#6976,#6978,#4054,.T.);
#8551=EDGE_CURVE('',#6979,#6977,#4055,.T.);
#8552=EDGE_CURVE('',#6978,#6979,#4056,.T.);
#8553=EDGE_CURVE('',#6978,#6980,#4057,.T.);
#8554=EDGE_CURVE('',#6981,#6979,#4058,.T.);
#8555=EDGE_CURVE('',#6980,#6981,#4059,.T.);
#8556=EDGE_CURVE('',#6980,#6982,#4060,.T.);
#8557=EDGE_CURVE('',#6983,#6981,#4061,.T.);
#8558=EDGE_CURVE('',#6982,#6983,#4062,.T.);
#8559=EDGE_CURVE('',#6982,#6984,#4063,.T.);
#8560=EDGE_CURVE('',#6985,#6983,#4064,.T.);
#8561=EDGE_CURVE('',#6984,#6985,#4065,.T.);
#8562=EDGE_CURVE('',#6984,#6986,#4066,.T.);
#8563=EDGE_CURVE('',#6987,#6985,#4067,.T.);
#8564=EDGE_CURVE('',#6986,#6987,#4068,.T.);
#8565=EDGE_CURVE('',#6986,#6988,#4069,.T.);
#8566=EDGE_CURVE('',#6989,#6987,#4070,.T.);
#8567=EDGE_CURVE('',#6988,#6989,#4071,.T.);
#8568=EDGE_CURVE('',#6988,#6990,#4072,.T.);
#8569=EDGE_CURVE('',#6991,#6989,#4073,.T.);
#8570=EDGE_CURVE('',#6990,#6991,#4074,.T.);
#8571=EDGE_CURVE('',#6990,#6992,#4075,.T.);
#8572=EDGE_CURVE('',#6993,#6991,#4076,.T.);
#8573=EDGE_CURVE('',#6992,#6993,#4077,.T.);
#8574=EDGE_CURVE('',#6992,#6994,#4078,.T.);
#8575=EDGE_CURVE('',#6995,#6993,#4079,.T.);
#8576=EDGE_CURVE('',#6994,#6995,#4080,.T.);
#8577=EDGE_CURVE('',#6994,#6996,#4081,.T.);
#8578=EDGE_CURVE('',#6997,#6995,#4082,.T.);
#8579=EDGE_CURVE('',#6996,#6997,#4083,.T.);
#8580=EDGE_CURVE('',#6996,#6998,#4084,.T.);
#8581=EDGE_CURVE('',#6999,#6997,#4085,.T.);
#8582=EDGE_CURVE('',#6998,#6999,#4086,.T.);
#8583=EDGE_CURVE('',#6998,#7000,#4087,.T.);
#8584=EDGE_CURVE('',#7001,#6999,#4088,.T.);
#8585=EDGE_CURVE('',#7000,#7001,#4089,.T.);
#8586=EDGE_CURVE('',#7000,#7002,#4090,.T.);
#8587=EDGE_CURVE('',#7003,#7001,#4091,.T.);
#8588=EDGE_CURVE('',#7002,#7003,#4092,.T.);
#8589=EDGE_CURVE('',#7002,#7004,#4093,.T.);
#8590=EDGE_CURVE('',#7005,#7003,#4094,.T.);
#8591=EDGE_CURVE('',#7004,#7005,#4095,.T.);
#8592=EDGE_CURVE('',#7004,#7006,#4096,.T.);
#8593=EDGE_CURVE('',#7007,#7005,#4097,.T.);
#8594=EDGE_CURVE('',#7006,#7007,#4098,.T.);
#8595=EDGE_CURVE('',#7006,#7008,#4099,.T.);
#8596=EDGE_CURVE('',#7009,#7007,#4100,.T.);
#8597=EDGE_CURVE('',#7008,#7009,#4101,.T.);
#8598=EDGE_CURVE('',#7008,#7010,#4102,.T.);
#8599=EDGE_CURVE('',#7011,#7009,#4103,.T.);
#8600=EDGE_CURVE('',#7010,#7011,#4104,.T.);
#8601=EDGE_CURVE('',#7010,#7012,#4105,.T.);
#8602=EDGE_CURVE('',#7013,#7011,#4106,.T.);
#8603=EDGE_CURVE('',#7012,#7013,#4107,.T.);
#8604=EDGE_CURVE('',#7012,#7014,#4108,.T.);
#8605=EDGE_CURVE('',#7015,#7013,#4109,.T.);
#8606=EDGE_CURVE('',#7014,#7015,#4110,.T.);
#8607=EDGE_CURVE('',#7014,#7016,#4111,.T.);
#8608=EDGE_CURVE('',#7017,#7015,#4112,.T.);
#8609=EDGE_CURVE('',#7016,#7017,#4113,.T.);
#8610=EDGE_CURVE('',#7016,#7018,#4114,.T.);
#8611=EDGE_CURVE('',#7019,#7017,#4115,.T.);
#8612=EDGE_CURVE('',#7018,#7019,#4116,.T.);
#8613=EDGE_CURVE('',#7018,#7020,#4117,.T.);
#8614=EDGE_CURVE('',#7021,#7019,#4118,.T.);
#8615=EDGE_CURVE('',#7020,#7021,#4119,.T.);
#8616=EDGE_CURVE('',#7020,#6766,#4120,.T.);
#8617=EDGE_CURVE('',#6768,#7021,#4121,.T.);
#10820=ORIENTED_EDGE('',*,*,#8222,.F.);
#10821=ORIENTED_EDGE('',*,*,#8223,.T.);
#10822=ORIENTED_EDGE('',*,*,#8224,.T.);
#10823=ORIENTED_EDGE('',*,*,#8223,.F.);
#10824=ORIENTED_EDGE('',*,*,#8224,.F.);
#10825=ORIENTED_EDGE('',*,*,#8225,.F.);
#10826=ORIENTED_EDGE('',*,*,#8226,.T.);
#10827=ORIENTED_EDGE('',*,*,#8227,.T.);
#10828=ORIENTED_EDGE('',*,*,#8226,.F.);
#10829=ORIENTED_EDGE('',*,*,#8227,.F.);
#10830=ORIENTED_EDGE('',*,*,#8228,.F.);
#10831=ORIENTED_EDGE('',*,*,#8229,.T.);
#10832=ORIENTED_EDGE('',*,*,#8230,.T.);
#10833=ORIENTED_EDGE('',*,*,#8229,.F.);
#10834=ORIENTED_EDGE('',*,*,#8230,.F.);
#10835=ORIENTED_EDGE('',*,*,#8231,.F.);
#10836=ORIENTED_EDGE('',*,*,#8232,.T.);
#10837=ORIENTED_EDGE('',*,*,#8233,.T.);
#10838=ORIENTED_EDGE('',*,*,#8232,.F.);
#10839=ORIENTED_EDGE('',*,*,#8233,.F.);
#10840=ORIENTED_EDGE('',*,*,#8234,.F.);
#10841=ORIENTED_EDGE('',*,*,#8235,.T.);
#10842=ORIENTED_EDGE('',*,*,#8236,.F.);
#10843=ORIENTED_EDGE('',*,*,#8237,.F.);
#10844=ORIENTED_EDGE('',*,*,#8238,.F.);
#10845=ORIENTED_EDGE('',*,*,#8237,.T.);
#10846=ORIENTED_EDGE('',*,*,#8239,.F.);
#10847=ORIENTED_EDGE('',*,*,#8240,.F.);
#10848=ORIENTED_EDGE('',*,*,#8222,.T.);
#10849=ORIENTED_EDGE('',*,*,#8225,.T.);
#10850=ORIENTED_EDGE('',*,*,#8228,.T.);
#10851=ORIENTED_EDGE('',*,*,#8231,.T.);
#10852=ORIENTED_EDGE('',*,*,#8241,.F.);
#10853=ORIENTED_EDGE('',*,*,#8240,.T.);
#10854=ORIENTED_EDGE('',*,*,#8242,.F.);
#10855=ORIENTED_EDGE('',*,*,#8243,.F.);
#10856=ORIENTED_EDGE('',*,*,#8244,.F.);
#10857=ORIENTED_EDGE('',*,*,#8243,.T.);
#10858=ORIENTED_EDGE('',*,*,#8245,.F.);
#10859=ORIENTED_EDGE('',*,*,#8246,.F.);
#10860=ORIENTED_EDGE('',*,*,#8247,.F.);
#10861=ORIENTED_EDGE('',*,*,#8246,.T.);
#10862=ORIENTED_EDGE('',*,*,#8248,.F.);
#10863=ORIENTED_EDGE('',*,*,#8249,.F.);
#10864=ORIENTED_EDGE('',*,*,#8250,.F.);
#10865=ORIENTED_EDGE('',*,*,#8249,.T.);
#10866=ORIENTED_EDGE('',*,*,#8251,.F.);
#10867=ORIENTED_EDGE('',*,*,#8252,.F.);
#10868=ORIENTED_EDGE('',*,*,#8253,.F.);
#10869=ORIENTED_EDGE('',*,*,#8252,.T.);
#10870=ORIENTED_EDGE('',*,*,#8254,.F.);
#10871=ORIENTED_EDGE('',*,*,#8255,.F.);
#10872=ORIENTED_EDGE('',*,*,#8256,.F.);
#10873=ORIENTED_EDGE('',*,*,#8255,.T.);
#10874=ORIENTED_EDGE('',*,*,#8257,.F.);
#10875=ORIENTED_EDGE('',*,*,#8258,.F.);
#10876=ORIENTED_EDGE('',*,*,#8259,.F.);
#10877=ORIENTED_EDGE('',*,*,#8258,.T.);
#10878=ORIENTED_EDGE('',*,*,#8260,.F.);
#10879=ORIENTED_EDGE('',*,*,#8261,.F.);
#10880=ORIENTED_EDGE('',*,*,#8262,.F.);
#10881=ORIENTED_EDGE('',*,*,#8261,.T.);
#10882=ORIENTED_EDGE('',*,*,#8263,.F.);
#10883=ORIENTED_EDGE('',*,*,#8264,.F.);
#10884=ORIENTED_EDGE('',*,*,#8265,.F.);
#10885=ORIENTED_EDGE('',*,*,#8264,.T.);
#10886=ORIENTED_EDGE('',*,*,#8266,.F.);
#10887=ORIENTED_EDGE('',*,*,#8267,.F.);
#10888=ORIENTED_EDGE('',*,*,#8268,.F.);
#10889=ORIENTED_EDGE('',*,*,#8267,.T.);
#10890=ORIENTED_EDGE('',*,*,#8269,.F.);
#10891=ORIENTED_EDGE('',*,*,#8270,.F.);
#10892=ORIENTED_EDGE('',*,*,#8271,.F.);
#10893=ORIENTED_EDGE('',*,*,#8270,.T.);
#10894=ORIENTED_EDGE('',*,*,#8272,.F.);
#10895=ORIENTED_EDGE('',*,*,#8273,.F.);
#10896=ORIENTED_EDGE('',*,*,#8274,.F.);
#10897=ORIENTED_EDGE('',*,*,#8273,.T.);
#10898=ORIENTED_EDGE('',*,*,#8275,.F.);
#10899=ORIENTED_EDGE('',*,*,#8276,.F.);
#10900=ORIENTED_EDGE('',*,*,#8277,.F.);
#10901=ORIENTED_EDGE('',*,*,#8276,.T.);
#10902=ORIENTED_EDGE('',*,*,#8278,.F.);
#10903=ORIENTED_EDGE('',*,*,#8279,.F.);
#10904=ORIENTED_EDGE('',*,*,#8280,.F.);
#10905=ORIENTED_EDGE('',*,*,#8279,.T.);
#10906=ORIENTED_EDGE('',*,*,#8281,.F.);
#10907=ORIENTED_EDGE('',*,*,#8282,.F.);
#10908=ORIENTED_EDGE('',*,*,#8283,.F.);
#10909=ORIENTED_EDGE('',*,*,#8282,.T.);
#10910=ORIENTED_EDGE('',*,*,#8284,.F.);
#10911=ORIENTED_EDGE('',*,*,#8285,.F.);
#10912=ORIENTED_EDGE('',*,*,#8286,.F.);
#10913=ORIENTED_EDGE('',*,*,#8285,.T.);
#10914=ORIENTED_EDGE('',*,*,#8287,.F.);
#10915=ORIENTED_EDGE('',*,*,#8288,.F.);
#10916=ORIENTED_EDGE('',*,*,#8289,.F.);
#10917=ORIENTED_EDGE('',*,*,#8288,.T.);
#10918=ORIENTED_EDGE('',*,*,#8290,.F.);
#10919=ORIENTED_EDGE('',*,*,#8291,.F.);
#10920=ORIENTED_EDGE('',*,*,#8292,.F.);
#10921=ORIENTED_EDGE('',*,*,#8291,.T.);
#10922=ORIENTED_EDGE('',*,*,#8293,.F.);
#10923=ORIENTED_EDGE('',*,*,#8294,.F.);
#10924=ORIENTED_EDGE('',*,*,#8295,.F.);
#10925=ORIENTED_EDGE('',*,*,#8294,.T.);
#10926=ORIENTED_EDGE('',*,*,#8296,.F.);
#10927=ORIENTED_EDGE('',*,*,#8297,.F.);
#10928=ORIENTED_EDGE('',*,*,#8298,.F.);
#10929=ORIENTED_EDGE('',*,*,#8297,.T.);
#10930=ORIENTED_EDGE('',*,*,#8299,.F.);
#10931=ORIENTED_EDGE('',*,*,#8300,.F.);
#10932=ORIENTED_EDGE('',*,*,#8301,.F.);
#10933=ORIENTED_EDGE('',*,*,#8300,.T.);
#10934=ORIENTED_EDGE('',*,*,#8302,.F.);
#10935=ORIENTED_EDGE('',*,*,#8303,.F.);
#10936=ORIENTED_EDGE('',*,*,#8304,.F.);
#10937=ORIENTED_EDGE('',*,*,#8303,.T.);
#10938=ORIENTED_EDGE('',*,*,#8305,.F.);
#10939=ORIENTED_EDGE('',*,*,#8306,.F.);
#10940=ORIENTED_EDGE('',*,*,#8307,.F.);
#10941=ORIENTED_EDGE('',*,*,#8306,.T.);
#10942=ORIENTED_EDGE('',*,*,#8308,.F.);
#10943=ORIENTED_EDGE('',*,*,#8309,.F.);
#10944=ORIENTED_EDGE('',*,*,#8310,.F.);
#10945=ORIENTED_EDGE('',*,*,#8309,.T.);
#10946=ORIENTED_EDGE('',*,*,#8311,.F.);
#10947=ORIENTED_EDGE('',*,*,#8312,.F.);
#10948=ORIENTED_EDGE('',*,*,#8313,.F.);
#10949=ORIENTED_EDGE('',*,*,#8312,.T.);
#10950=ORIENTED_EDGE('',*,*,#8314,.F.);
#10951=ORIENTED_EDGE('',*,*,#8315,.F.);
#10952=ORIENTED_EDGE('',*,*,#8316,.F.);
#10953=ORIENTED_EDGE('',*,*,#8315,.T.);
#10954=ORIENTED_EDGE('',*,*,#8317,.F.);
#10955=ORIENTED_EDGE('',*,*,#8318,.F.);
#10956=ORIENTED_EDGE('',*,*,#8319,.F.);
#10957=ORIENTED_EDGE('',*,*,#8318,.T.);
#10958=ORIENTED_EDGE('',*,*,#8320,.F.);
#10959=ORIENTED_EDGE('',*,*,#8321,.F.);
#10960=ORIENTED_EDGE('',*,*,#8322,.F.);
#10961=ORIENTED_EDGE('',*,*,#8321,.T.);
#10962=ORIENTED_EDGE('',*,*,#8323,.F.);
#10963=ORIENTED_EDGE('',*,*,#8324,.F.);
#10964=ORIENTED_EDGE('',*,*,#8325,.F.);
#10965=ORIENTED_EDGE('',*,*,#8324,.T.);
#10966=ORIENTED_EDGE('',*,*,#8326,.F.);
#10967=ORIENTED_EDGE('',*,*,#8327,.F.);
#10968=ORIENTED_EDGE('',*,*,#8328,.F.);
#10969=ORIENTED_EDGE('',*,*,#8327,.T.);
#10970=ORIENTED_EDGE('',*,*,#8329,.F.);
#10971=ORIENTED_EDGE('',*,*,#8330,.F.);
#10972=ORIENTED_EDGE('',*,*,#8331,.F.);
#10973=ORIENTED_EDGE('',*,*,#8330,.T.);
#10974=ORIENTED_EDGE('',*,*,#8332,.F.);
#10975=ORIENTED_EDGE('',*,*,#8333,.F.);
#10976=ORIENTED_EDGE('',*,*,#8334,.F.);
#10977=ORIENTED_EDGE('',*,*,#8333,.T.);
#10978=ORIENTED_EDGE('',*,*,#8335,.F.);
#10979=ORIENTED_EDGE('',*,*,#8336,.F.);
#10980=ORIENTED_EDGE('',*,*,#8337,.F.);
#10981=ORIENTED_EDGE('',*,*,#8336,.T.);
#10982=ORIENTED_EDGE('',*,*,#8338,.F.);
#10983=ORIENTED_EDGE('',*,*,#8339,.F.);
#10984=ORIENTED_EDGE('',*,*,#8340,.F.);
#10985=ORIENTED_EDGE('',*,*,#8339,.T.);
#10986=ORIENTED_EDGE('',*,*,#8341,.F.);
#10987=ORIENTED_EDGE('',*,*,#8342,.F.);
#10988=ORIENTED_EDGE('',*,*,#8343,.F.);
#10989=ORIENTED_EDGE('',*,*,#8342,.T.);
#10990=ORIENTED_EDGE('',*,*,#8344,.F.);
#10991=ORIENTED_EDGE('',*,*,#8345,.F.);
#10992=ORIENTED_EDGE('',*,*,#8346,.F.);
#10993=ORIENTED_EDGE('',*,*,#8345,.T.);
#10994=ORIENTED_EDGE('',*,*,#8347,.F.);
#10995=ORIENTED_EDGE('',*,*,#8348,.F.);
#10996=ORIENTED_EDGE('',*,*,#8349,.F.);
#10997=ORIENTED_EDGE('',*,*,#8348,.T.);
#10998=ORIENTED_EDGE('',*,*,#8350,.F.);
#10999=ORIENTED_EDGE('',*,*,#8351,.F.);
#11000=ORIENTED_EDGE('',*,*,#8352,.F.);
#11001=ORIENTED_EDGE('',*,*,#8351,.T.);
#11002=ORIENTED_EDGE('',*,*,#8353,.F.);
#11003=ORIENTED_EDGE('',*,*,#8354,.F.);
#11004=ORIENTED_EDGE('',*,*,#8355,.F.);
#11005=ORIENTED_EDGE('',*,*,#8354,.T.);
#11006=ORIENTED_EDGE('',*,*,#8356,.F.);
#11007=ORIENTED_EDGE('',*,*,#8357,.F.);
#11008=ORIENTED_EDGE('',*,*,#8358,.F.);
#11009=ORIENTED_EDGE('',*,*,#8357,.T.);
#11010=ORIENTED_EDGE('',*,*,#8359,.F.);
#11011=ORIENTED_EDGE('',*,*,#8360,.F.);
#11012=ORIENTED_EDGE('',*,*,#8361,.F.);
#11013=ORIENTED_EDGE('',*,*,#8360,.T.);
#11014=ORIENTED_EDGE('',*,*,#8362,.F.);
#11015=ORIENTED_EDGE('',*,*,#8363,.F.);
#11016=ORIENTED_EDGE('',*,*,#8364,.F.);
#11017=ORIENTED_EDGE('',*,*,#8363,.T.);
#11018=ORIENTED_EDGE('',*,*,#8365,.F.);
#11019=ORIENTED_EDGE('',*,*,#8366,.F.);
#11020=ORIENTED_EDGE('',*,*,#8367,.F.);
#11021=ORIENTED_EDGE('',*,*,#8366,.T.);
#11022=ORIENTED_EDGE('',*,*,#8368,.F.);
#11023=ORIENTED_EDGE('',*,*,#8369,.F.);
#11024=ORIENTED_EDGE('',*,*,#8370,.F.);
#11025=ORIENTED_EDGE('',*,*,#8369,.T.);
#11026=ORIENTED_EDGE('',*,*,#8371,.F.);
#11027=ORIENTED_EDGE('',*,*,#8372,.F.);
#11028=ORIENTED_EDGE('',*,*,#8373,.F.);
#11029=ORIENTED_EDGE('',*,*,#8372,.T.);
#11030=ORIENTED_EDGE('',*,*,#8374,.F.);
#11031=ORIENTED_EDGE('',*,*,#8375,.F.);
#11032=ORIENTED_EDGE('',*,*,#8376,.F.);
#11033=ORIENTED_EDGE('',*,*,#8375,.T.);
#11034=ORIENTED_EDGE('',*,*,#8377,.F.);
#11035=ORIENTED_EDGE('',*,*,#8378,.F.);
#11036=ORIENTED_EDGE('',*,*,#8379,.F.);
#11037=ORIENTED_EDGE('',*,*,#8378,.T.);
#11038=ORIENTED_EDGE('',*,*,#8380,.F.);
#11039=ORIENTED_EDGE('',*,*,#8381,.F.);
#11040=ORIENTED_EDGE('',*,*,#8382,.F.);
#11041=ORIENTED_EDGE('',*,*,#8381,.T.);
#11042=ORIENTED_EDGE('',*,*,#8383,.F.);
#11043=ORIENTED_EDGE('',*,*,#8384,.F.);
#11044=ORIENTED_EDGE('',*,*,#8385,.F.);
#11045=ORIENTED_EDGE('',*,*,#8384,.T.);
#11046=ORIENTED_EDGE('',*,*,#8386,.F.);
#11047=ORIENTED_EDGE('',*,*,#8387,.F.);
#11048=ORIENTED_EDGE('',*,*,#8388,.F.);
#11049=ORIENTED_EDGE('',*,*,#8387,.T.);
#11050=ORIENTED_EDGE('',*,*,#8389,.F.);
#11051=ORIENTED_EDGE('',*,*,#8390,.F.);
#11052=ORIENTED_EDGE('',*,*,#8391,.F.);
#11053=ORIENTED_EDGE('',*,*,#8390,.T.);
#11054=ORIENTED_EDGE('',*,*,#8392,.F.);
#11055=ORIENTED_EDGE('',*,*,#8393,.F.);
#11056=ORIENTED_EDGE('',*,*,#8394,.F.);
#11057=ORIENTED_EDGE('',*,*,#8393,.T.);
#11058=ORIENTED_EDGE('',*,*,#8395,.F.);
#11059=ORIENTED_EDGE('',*,*,#8396,.F.);
#11060=ORIENTED_EDGE('',*,*,#8397,.F.);
#11061=ORIENTED_EDGE('',*,*,#8396,.T.);
#11062=ORIENTED_EDGE('',*,*,#8398,.F.);
#11063=ORIENTED_EDGE('',*,*,#8399,.F.);
#11064=ORIENTED_EDGE('',*,*,#8400,.F.);
#11065=ORIENTED_EDGE('',*,*,#8399,.T.);
#11066=ORIENTED_EDGE('',*,*,#8401,.F.);
#11067=ORIENTED_EDGE('',*,*,#8402,.F.);
#11068=ORIENTED_EDGE('',*,*,#8403,.F.);
#11069=ORIENTED_EDGE('',*,*,#8402,.T.);
#11070=ORIENTED_EDGE('',*,*,#8404,.F.);
#11071=ORIENTED_EDGE('',*,*,#8405,.F.);
#11072=ORIENTED_EDGE('',*,*,#8406,.F.);
#11073=ORIENTED_EDGE('',*,*,#8405,.T.);
#11074=ORIENTED_EDGE('',*,*,#8407,.F.);
#11075=ORIENTED_EDGE('',*,*,#8408,.F.);
#11076=ORIENTED_EDGE('',*,*,#8409,.F.);
#11077=ORIENTED_EDGE('',*,*,#8408,.T.);
#11078=ORIENTED_EDGE('',*,*,#8410,.F.);
#11079=ORIENTED_EDGE('',*,*,#8411,.F.);
#11080=ORIENTED_EDGE('',*,*,#8412,.F.);
#11081=ORIENTED_EDGE('',*,*,#8411,.T.);
#11082=ORIENTED_EDGE('',*,*,#8413,.F.);
#11083=ORIENTED_EDGE('',*,*,#8414,.F.);
#11084=ORIENTED_EDGE('',*,*,#8415,.F.);
#11085=ORIENTED_EDGE('',*,*,#8414,.T.);
#11086=ORIENTED_EDGE('',*,*,#8416,.F.);
#11087=ORIENTED_EDGE('',*,*,#8417,.F.);
#11088=ORIENTED_EDGE('',*,*,#8418,.F.);
#11089=ORIENTED_EDGE('',*,*,#8417,.T.);
#11090=ORIENTED_EDGE('',*,*,#8419,.F.);
#11091=ORIENTED_EDGE('',*,*,#8420,.F.);
#11092=ORIENTED_EDGE('',*,*,#8421,.F.);
#11093=ORIENTED_EDGE('',*,*,#8420,.T.);
#11094=ORIENTED_EDGE('',*,*,#8422,.F.);
#11095=ORIENTED_EDGE('',*,*,#8423,.F.);
#11096=ORIENTED_EDGE('',*,*,#8424,.F.);
#11097=ORIENTED_EDGE('',*,*,#8423,.T.);
#11098=ORIENTED_EDGE('',*,*,#8425,.F.);
#11099=ORIENTED_EDGE('',*,*,#8426,.F.);
#11100=ORIENTED_EDGE('',*,*,#8427,.F.);
#11101=ORIENTED_EDGE('',*,*,#8426,.T.);
#11102=ORIENTED_EDGE('',*,*,#8428,.F.);
#11103=ORIENTED_EDGE('',*,*,#8429,.F.);
#11104=ORIENTED_EDGE('',*,*,#8430,.F.);
#11105=ORIENTED_EDGE('',*,*,#8429,.T.);
#11106=ORIENTED_EDGE('',*,*,#8431,.F.);
#11107=ORIENTED_EDGE('',*,*,#8432,.F.);
#11108=ORIENTED_EDGE('',*,*,#8433,.F.);
#11109=ORIENTED_EDGE('',*,*,#8432,.T.);
#11110=ORIENTED_EDGE('',*,*,#8434,.F.);
#11111=ORIENTED_EDGE('',*,*,#8435,.F.);
#11112=ORIENTED_EDGE('',*,*,#8436,.F.);
#11113=ORIENTED_EDGE('',*,*,#8435,.T.);
#11114=ORIENTED_EDGE('',*,*,#8437,.F.);
#11115=ORIENTED_EDGE('',*,*,#8438,.F.);
#11116=ORIENTED_EDGE('',*,*,#8439,.F.);
#11117=ORIENTED_EDGE('',*,*,#8438,.T.);
#11118=ORIENTED_EDGE('',*,*,#8440,.F.);
#11119=ORIENTED_EDGE('',*,*,#8441,.F.);
#11120=ORIENTED_EDGE('',*,*,#8442,.F.);
#11121=ORIENTED_EDGE('',*,*,#8441,.T.);
#11122=ORIENTED_EDGE('',*,*,#8443,.F.);
#11123=ORIENTED_EDGE('',*,*,#8444,.F.);
#11124=ORIENTED_EDGE('',*,*,#8445,.F.);
#11125=ORIENTED_EDGE('',*,*,#8444,.T.);
#11126=ORIENTED_EDGE('',*,*,#8446,.F.);
#11127=ORIENTED_EDGE('',*,*,#8447,.F.);
#11128=ORIENTED_EDGE('',*,*,#8448,.F.);
#11129=ORIENTED_EDGE('',*,*,#8447,.T.);
#11130=ORIENTED_EDGE('',*,*,#8449,.F.);
#11131=ORIENTED_EDGE('',*,*,#8450,.F.);
#11132=ORIENTED_EDGE('',*,*,#8451,.F.);
#11133=ORIENTED_EDGE('',*,*,#8450,.T.);
#11134=ORIENTED_EDGE('',*,*,#8452,.F.);
#11135=ORIENTED_EDGE('',*,*,#8453,.F.);
#11136=ORIENTED_EDGE('',*,*,#8454,.F.);
#11137=ORIENTED_EDGE('',*,*,#8453,.T.);
#11138=ORIENTED_EDGE('',*,*,#8455,.F.);
#11139=ORIENTED_EDGE('',*,*,#8456,.F.);
#11140=ORIENTED_EDGE('',*,*,#8457,.F.);
#11141=ORIENTED_EDGE('',*,*,#8456,.T.);
#11142=ORIENTED_EDGE('',*,*,#8458,.F.);
#11143=ORIENTED_EDGE('',*,*,#8459,.F.);
#11144=ORIENTED_EDGE('',*,*,#8460,.F.);
#11145=ORIENTED_EDGE('',*,*,#8459,.T.);
#11146=ORIENTED_EDGE('',*,*,#8461,.F.);
#11147=ORIENTED_EDGE('',*,*,#8462,.F.);
#11148=ORIENTED_EDGE('',*,*,#8463,.F.);
#11149=ORIENTED_EDGE('',*,*,#8462,.T.);
#11150=ORIENTED_EDGE('',*,*,#8464,.F.);
#11151=ORIENTED_EDGE('',*,*,#8465,.F.);
#11152=ORIENTED_EDGE('',*,*,#8466,.F.);
#11153=ORIENTED_EDGE('',*,*,#8465,.T.);
#11154=ORIENTED_EDGE('',*,*,#8467,.F.);
#11155=ORIENTED_EDGE('',*,*,#8468,.F.);
#11156=ORIENTED_EDGE('',*,*,#8469,.F.);
#11157=ORIENTED_EDGE('',*,*,#8468,.T.);
#11158=ORIENTED_EDGE('',*,*,#8470,.F.);
#11159=ORIENTED_EDGE('',*,*,#8471,.F.);
#11160=ORIENTED_EDGE('',*,*,#8472,.F.);
#11161=ORIENTED_EDGE('',*,*,#8471,.T.);
#11162=ORIENTED_EDGE('',*,*,#8473,.F.);
#11163=ORIENTED_EDGE('',*,*,#8474,.F.);
#11164=ORIENTED_EDGE('',*,*,#8475,.F.);
#11165=ORIENTED_EDGE('',*,*,#8474,.T.);
#11166=ORIENTED_EDGE('',*,*,#8476,.F.);
#11167=ORIENTED_EDGE('',*,*,#8477,.F.);
#11168=ORIENTED_EDGE('',*,*,#8478,.F.);
#11169=ORIENTED_EDGE('',*,*,#8477,.T.);
#11170=ORIENTED_EDGE('',*,*,#8479,.F.);
#11171=ORIENTED_EDGE('',*,*,#8480,.F.);
#11172=ORIENTED_EDGE('',*,*,#8481,.F.);
#11173=ORIENTED_EDGE('',*,*,#8480,.T.);
#11174=ORIENTED_EDGE('',*,*,#8482,.F.);
#11175=ORIENTED_EDGE('',*,*,#8483,.F.);
#11176=ORIENTED_EDGE('',*,*,#8484,.F.);
#11177=ORIENTED_EDGE('',*,*,#8483,.T.);
#11178=ORIENTED_EDGE('',*,*,#8485,.F.);
#11179=ORIENTED_EDGE('',*,*,#8486,.F.);
#11180=ORIENTED_EDGE('',*,*,#8487,.F.);
#11181=ORIENTED_EDGE('',*,*,#8486,.T.);
#11182=ORIENTED_EDGE('',*,*,#8488,.F.);
#11183=ORIENTED_EDGE('',*,*,#8489,.F.);
#11184=ORIENTED_EDGE('',*,*,#8490,.F.);
#11185=ORIENTED_EDGE('',*,*,#8489,.T.);
#11186=ORIENTED_EDGE('',*,*,#8491,.F.);
#11187=ORIENTED_EDGE('',*,*,#8492,.F.);
#11188=ORIENTED_EDGE('',*,*,#8493,.F.);
#11189=ORIENTED_EDGE('',*,*,#8492,.T.);
#11190=ORIENTED_EDGE('',*,*,#8494,.F.);
#11191=ORIENTED_EDGE('',*,*,#8495,.F.);
#11192=ORIENTED_EDGE('',*,*,#8496,.F.);
#11193=ORIENTED_EDGE('',*,*,#8495,.T.);
#11194=ORIENTED_EDGE('',*,*,#8497,.F.);
#11195=ORIENTED_EDGE('',*,*,#8498,.F.);
#11196=ORIENTED_EDGE('',*,*,#8499,.F.);
#11197=ORIENTED_EDGE('',*,*,#8498,.T.);
#11198=ORIENTED_EDGE('',*,*,#8500,.F.);
#11199=ORIENTED_EDGE('',*,*,#8501,.F.);
#11200=ORIENTED_EDGE('',*,*,#8502,.F.);
#11201=ORIENTED_EDGE('',*,*,#8501,.T.);
#11202=ORIENTED_EDGE('',*,*,#8503,.F.);
#11203=ORIENTED_EDGE('',*,*,#8504,.F.);
#11204=ORIENTED_EDGE('',*,*,#8505,.F.);
#11205=ORIENTED_EDGE('',*,*,#8504,.T.);
#11206=ORIENTED_EDGE('',*,*,#8506,.F.);
#11207=ORIENTED_EDGE('',*,*,#8507,.F.);
#11208=ORIENTED_EDGE('',*,*,#8508,.F.);
#11209=ORIENTED_EDGE('',*,*,#8507,.T.);
#11210=ORIENTED_EDGE('',*,*,#8509,.F.);
#11211=ORIENTED_EDGE('',*,*,#8510,.F.);
#11212=ORIENTED_EDGE('',*,*,#8511,.F.);
#11213=ORIENTED_EDGE('',*,*,#8510,.T.);
#11214=ORIENTED_EDGE('',*,*,#8512,.F.);
#11215=ORIENTED_EDGE('',*,*,#8513,.F.);
#11216=ORIENTED_EDGE('',*,*,#8514,.F.);
#11217=ORIENTED_EDGE('',*,*,#8513,.T.);
#11218=ORIENTED_EDGE('',*,*,#8515,.F.);
#11219=ORIENTED_EDGE('',*,*,#8516,.F.);
#11220=ORIENTED_EDGE('',*,*,#8517,.F.);
#11221=ORIENTED_EDGE('',*,*,#8516,.T.);
#11222=ORIENTED_EDGE('',*,*,#8518,.F.);
#11223=ORIENTED_EDGE('',*,*,#8519,.F.);
#11224=ORIENTED_EDGE('',*,*,#8520,.F.);
#11225=ORIENTED_EDGE('',*,*,#8519,.T.);
#11226=ORIENTED_EDGE('',*,*,#8521,.F.);
#11227=ORIENTED_EDGE('',*,*,#8522,.F.);
#11228=ORIENTED_EDGE('',*,*,#8523,.F.);
#11229=ORIENTED_EDGE('',*,*,#8522,.T.);
#11230=ORIENTED_EDGE('',*,*,#8524,.F.);
#11231=ORIENTED_EDGE('',*,*,#8525,.F.);
#11232=ORIENTED_EDGE('',*,*,#8526,.F.);
#11233=ORIENTED_EDGE('',*,*,#8525,.T.);
#11234=ORIENTED_EDGE('',*,*,#8527,.F.);
#11235=ORIENTED_EDGE('',*,*,#8528,.F.);
#11236=ORIENTED_EDGE('',*,*,#8529,.F.);
#11237=ORIENTED_EDGE('',*,*,#8528,.T.);
#11238=ORIENTED_EDGE('',*,*,#8530,.F.);
#11239=ORIENTED_EDGE('',*,*,#8531,.F.);
#11240=ORIENTED_EDGE('',*,*,#8532,.F.);
#11241=ORIENTED_EDGE('',*,*,#8531,.T.);
#11242=ORIENTED_EDGE('',*,*,#8533,.F.);
#11243=ORIENTED_EDGE('',*,*,#8534,.F.);
#11244=ORIENTED_EDGE('',*,*,#8535,.F.);
#11245=ORIENTED_EDGE('',*,*,#8534,.T.);
#11246=ORIENTED_EDGE('',*,*,#8536,.F.);
#11247=ORIENTED_EDGE('',*,*,#8537,.F.);
#11248=ORIENTED_EDGE('',*,*,#8538,.F.);
#11249=ORIENTED_EDGE('',*,*,#8537,.T.);
#11250=ORIENTED_EDGE('',*,*,#8539,.F.);
#11251=ORIENTED_EDGE('',*,*,#8540,.F.);
#11252=ORIENTED_EDGE('',*,*,#8541,.F.);
#11253=ORIENTED_EDGE('',*,*,#8540,.T.);
#11254=ORIENTED_EDGE('',*,*,#8542,.F.);
#11255=ORIENTED_EDGE('',*,*,#8543,.F.);
#11256=ORIENTED_EDGE('',*,*,#8544,.F.);
#11257=ORIENTED_EDGE('',*,*,#8543,.T.);
#11258=ORIENTED_EDGE('',*,*,#8545,.F.);
#11259=ORIENTED_EDGE('',*,*,#8546,.F.);
#11260=ORIENTED_EDGE('',*,*,#8547,.F.);
#11261=ORIENTED_EDGE('',*,*,#8546,.T.);
#11262=ORIENTED_EDGE('',*,*,#8548,.F.);
#11263=ORIENTED_EDGE('',*,*,#8549,.F.);
#11264=ORIENTED_EDGE('',*,*,#8550,.F.);
#11265=ORIENTED_EDGE('',*,*,#8549,.T.);
#11266=ORIENTED_EDGE('',*,*,#8551,.F.);
#11267=ORIENTED_EDGE('',*,*,#8552,.F.);
#11268=ORIENTED_EDGE('',*,*,#8553,.F.);
#11269=ORIENTED_EDGE('',*,*,#8552,.T.);
#11270=ORIENTED_EDGE('',*,*,#8554,.F.);
#11271=ORIENTED_EDGE('',*,*,#8555,.F.);
#11272=ORIENTED_EDGE('',*,*,#8556,.F.);
#11273=ORIENTED_EDGE('',*,*,#8555,.T.);
#11274=ORIENTED_EDGE('',*,*,#8557,.F.);
#11275=ORIENTED_EDGE('',*,*,#8558,.F.);
#11276=ORIENTED_EDGE('',*,*,#8559,.F.);
#11277=ORIENTED_EDGE('',*,*,#8558,.T.);
#11278=ORIENTED_EDGE('',*,*,#8560,.F.);
#11279=ORIENTED_EDGE('',*,*,#8561,.F.);
#11280=ORIENTED_EDGE('',*,*,#8562,.F.);
#11281=ORIENTED_EDGE('',*,*,#8561,.T.);
#11282=ORIENTED_EDGE('',*,*,#8563,.F.);
#11283=ORIENTED_EDGE('',*,*,#8564,.F.);
#11284=ORIENTED_EDGE('',*,*,#8565,.F.);
#11285=ORIENTED_EDGE('',*,*,#8564,.T.);
#11286=ORIENTED_EDGE('',*,*,#8566,.F.);
#11287=ORIENTED_EDGE('',*,*,#8567,.F.);
#11288=ORIENTED_EDGE('',*,*,#8568,.F.);
#11289=ORIENTED_EDGE('',*,*,#8567,.T.);
#11290=ORIENTED_EDGE('',*,*,#8569,.F.);
#11291=ORIENTED_EDGE('',*,*,#8570,.F.);
#11292=ORIENTED_EDGE('',*,*,#8571,.F.);
#11293=ORIENTED_EDGE('',*,*,#8570,.T.);
#11294=ORIENTED_EDGE('',*,*,#8572,.F.);
#11295=ORIENTED_EDGE('',*,*,#8573,.F.);
#11296=ORIENTED_EDGE('',*,*,#8574,.F.);
#11297=ORIENTED_EDGE('',*,*,#8573,.T.);
#11298=ORIENTED_EDGE('',*,*,#8575,.F.);
#11299=ORIENTED_EDGE('',*,*,#8576,.F.);
#11300=ORIENTED_EDGE('',*,*,#8577,.F.);
#11301=ORIENTED_EDGE('',*,*,#8576,.T.);
#11302=ORIENTED_EDGE('',*,*,#8578,.F.);
#11303=ORIENTED_EDGE('',*,*,#8579,.F.);
#11304=ORIENTED_EDGE('',*,*,#8580,.F.);
#11305=ORIENTED_EDGE('',*,*,#8579,.T.);
#11306=ORIENTED_EDGE('',*,*,#8581,.F.);
#11307=ORIENTED_EDGE('',*,*,#8582,.F.);
#11308=ORIENTED_EDGE('',*,*,#8583,.F.);
#11309=ORIENTED_EDGE('',*,*,#8582,.T.);
#11310=ORIENTED_EDGE('',*,*,#8584,.F.);
#11311=ORIENTED_EDGE('',*,*,#8585,.F.);
#11312=ORIENTED_EDGE('',*,*,#8586,.F.);
#11313=ORIENTED_EDGE('',*,*,#8585,.T.);
#11314=ORIENTED_EDGE('',*,*,#8587,.F.);
#11315=ORIENTED_EDGE('',*,*,#8588,.F.);
#11316=ORIENTED_EDGE('',*,*,#8589,.F.);
#11317=ORIENTED_EDGE('',*,*,#8588,.T.);
#11318=ORIENTED_EDGE('',*,*,#8590,.F.);
#11319=ORIENTED_EDGE('',*,*,#8591,.F.);
#11320=ORIENTED_EDGE('',*,*,#8592,.F.);
#11321=ORIENTED_EDGE('',*,*,#8591,.T.);
#11322=ORIENTED_EDGE('',*,*,#8593,.F.);
#11323=ORIENTED_EDGE('',*,*,#8594,.F.);
#11324=ORIENTED_EDGE('',*,*,#8595,.F.);
#11325=ORIENTED_EDGE('',*,*,#8594,.T.);
#11326=ORIENTED_EDGE('',*,*,#8596,.F.);
#11327=ORIENTED_EDGE('',*,*,#8597,.F.);
#11328=ORIENTED_EDGE('',*,*,#8598,.F.);
#11329=ORIENTED_EDGE('',*,*,#8597,.T.);
#11330=ORIENTED_EDGE('',*,*,#8599,.F.);
#11331=ORIENTED_EDGE('',*,*,#8600,.F.);
#11332=ORIENTED_EDGE('',*,*,#8601,.F.);
#11333=ORIENTED_EDGE('',*,*,#8600,.T.);
#11334=ORIENTED_EDGE('',*,*,#8602,.F.);
#11335=ORIENTED_EDGE('',*,*,#8603,.F.);
#11336=ORIENTED_EDGE('',*,*,#8604,.F.);
#11337=ORIENTED_EDGE('',*,*,#8603,.T.);
#11338=ORIENTED_EDGE('',*,*,#8605,.F.);
#11339=ORIENTED_EDGE('',*,*,#8606,.F.);
#11340=ORIENTED_EDGE('',*,*,#8607,.F.);
#11341=ORIENTED_EDGE('',*,*,#8606,.T.);
#11342=ORIENTED_EDGE('',*,*,#8608,.F.);
#11343=ORIENTED_EDGE('',*,*,#8609,.F.);
#11344=ORIENTED_EDGE('',*,*,#8610,.F.);
#11345=ORIENTED_EDGE('',*,*,#8609,.T.);
#11346=ORIENTED_EDGE('',*,*,#8611,.F.);
#11347=ORIENTED_EDGE('',*,*,#8612,.F.);
#11348=ORIENTED_EDGE('',*,*,#8613,.F.);
#11349=ORIENTED_EDGE('',*,*,#8612,.T.);
#11350=ORIENTED_EDGE('',*,*,#8614,.F.);
#11351=ORIENTED_EDGE('',*,*,#8615,.F.);
#11352=ORIENTED_EDGE('',*,*,#8616,.F.);
#11353=ORIENTED_EDGE('',*,*,#8615,.T.);
#11354=ORIENTED_EDGE('',*,*,#8617,.F.);
#11355=ORIENTED_EDGE('',*,*,#8235,.F.);
#11356=ORIENTED_EDGE('',*,*,#8617,.T.);
#11357=ORIENTED_EDGE('',*,*,#8614,.T.);
#11358=ORIENTED_EDGE('',*,*,#8611,.T.);
#11359=ORIENTED_EDGE('',*,*,#8608,.T.);
#11360=ORIENTED_EDGE('',*,*,#8605,.T.);
#11361=ORIENTED_EDGE('',*,*,#8602,.T.);
#11362=ORIENTED_EDGE('',*,*,#8599,.T.);
#11363=ORIENTED_EDGE('',*,*,#8596,.T.);
#11364=ORIENTED_EDGE('',*,*,#8593,.T.);
#11365=ORIENTED_EDGE('',*,*,#8590,.T.);
#11366=ORIENTED_EDGE('',*,*,#8587,.T.);
#11367=ORIENTED_EDGE('',*,*,#8584,.T.);
#11368=ORIENTED_EDGE('',*,*,#8581,.T.);
#11369=ORIENTED_EDGE('',*,*,#8578,.T.);
#11370=ORIENTED_EDGE('',*,*,#8575,.T.);
#11371=ORIENTED_EDGE('',*,*,#8572,.T.);
#11372=ORIENTED_EDGE('',*,*,#8569,.T.);
#11373=ORIENTED_EDGE('',*,*,#8566,.T.);
#11374=ORIENTED_EDGE('',*,*,#8563,.T.);
#11375=ORIENTED_EDGE('',*,*,#8560,.T.);
#11376=ORIENTED_EDGE('',*,*,#8557,.T.);
#11377=ORIENTED_EDGE('',*,*,#8554,.T.);
#11378=ORIENTED_EDGE('',*,*,#8551,.T.);
#11379=ORIENTED_EDGE('',*,*,#8548,.T.);
#11380=ORIENTED_EDGE('',*,*,#8545,.T.);
#11381=ORIENTED_EDGE('',*,*,#8542,.T.);
#11382=ORIENTED_EDGE('',*,*,#8539,.T.);
#11383=ORIENTED_EDGE('',*,*,#8536,.T.);
#11384=ORIENTED_EDGE('',*,*,#8533,.T.);
#11385=ORIENTED_EDGE('',*,*,#8530,.T.);
#11386=ORIENTED_EDGE('',*,*,#8527,.T.);
#11387=ORIENTED_EDGE('',*,*,#8524,.T.);
#11388=ORIENTED_EDGE('',*,*,#8521,.T.);
#11389=ORIENTED_EDGE('',*,*,#8518,.T.);
#11390=ORIENTED_EDGE('',*,*,#8515,.T.);
#11391=ORIENTED_EDGE('',*,*,#8512,.T.);
#11392=ORIENTED_EDGE('',*,*,#8509,.T.);
#11393=ORIENTED_EDGE('',*,*,#8506,.T.);
#11394=ORIENTED_EDGE('',*,*,#8503,.T.);
#11395=ORIENTED_EDGE('',*,*,#8500,.T.);
#11396=ORIENTED_EDGE('',*,*,#8497,.T.);
#11397=ORIENTED_EDGE('',*,*,#8494,.T.);
#11398=ORIENTED_EDGE('',*,*,#8491,.T.);
#11399=ORIENTED_EDGE('',*,*,#8488,.T.);
#11400=ORIENTED_EDGE('',*,*,#8485,.T.);
#11401=ORIENTED_EDGE('',*,*,#8482,.T.);
#11402=ORIENTED_EDGE('',*,*,#8479,.T.);
#11403=ORIENTED_EDGE('',*,*,#8476,.T.);
#11404=ORIENTED_EDGE('',*,*,#8473,.T.);
#11405=ORIENTED_EDGE('',*,*,#8470,.T.);
#11406=ORIENTED_EDGE('',*,*,#8467,.T.);
#11407=ORIENTED_EDGE('',*,*,#8464,.T.);
#11408=ORIENTED_EDGE('',*,*,#8461,.T.);
#11409=ORIENTED_EDGE('',*,*,#8458,.T.);
#11410=ORIENTED_EDGE('',*,*,#8455,.T.);
#11411=ORIENTED_EDGE('',*,*,#8452,.T.);
#11412=ORIENTED_EDGE('',*,*,#8449,.T.);
#11413=ORIENTED_EDGE('',*,*,#8446,.T.);
#11414=ORIENTED_EDGE('',*,*,#8443,.T.);
#11415=ORIENTED_EDGE('',*,*,#8440,.T.);
#11416=ORIENTED_EDGE('',*,*,#8437,.T.);
#11417=ORIENTED_EDGE('',*,*,#8434,.T.);
#11418=ORIENTED_EDGE('',*,*,#8431,.T.);
#11419=ORIENTED_EDGE('',*,*,#8428,.T.);
#11420=ORIENTED_EDGE('',*,*,#8425,.T.);
#11421=ORIENTED_EDGE('',*,*,#8422,.T.);
#11422=ORIENTED_EDGE('',*,*,#8419,.T.);
#11423=ORIENTED_EDGE('',*,*,#8416,.T.);
#11424=ORIENTED_EDGE('',*,*,#8413,.T.);
#11425=ORIENTED_EDGE('',*,*,#8410,.T.);
#11426=ORIENTED_EDGE('',*,*,#8407,.T.);
#11427=ORIENTED_EDGE('',*,*,#8404,.T.);
#11428=ORIENTED_EDGE('',*,*,#8401,.T.);
#11429=ORIENTED_EDGE('',*,*,#8398,.T.);
#11430=ORIENTED_EDGE('',*,*,#8395,.T.);
#11431=ORIENTED_EDGE('',*,*,#8392,.T.);
#11432=ORIENTED_EDGE('',*,*,#8389,.T.);
#11433=ORIENTED_EDGE('',*,*,#8386,.T.);
#11434=ORIENTED_EDGE('',*,*,#8383,.T.);
#11435=ORIENTED_EDGE('',*,*,#8380,.T.);
#11436=ORIENTED_EDGE('',*,*,#8377,.T.);
#11437=ORIENTED_EDGE('',*,*,#8374,.T.);
#11438=ORIENTED_EDGE('',*,*,#8371,.T.);
#11439=ORIENTED_EDGE('',*,*,#8368,.T.);
#11440=ORIENTED_EDGE('',*,*,#8365,.T.);
#11441=ORIENTED_EDGE('',*,*,#8362,.T.);
#11442=ORIENTED_EDGE('',*,*,#8359,.T.);
#11443=ORIENTED_EDGE('',*,*,#8356,.T.);
#11444=ORIENTED_EDGE('',*,*,#8353,.T.);
#11445=ORIENTED_EDGE('',*,*,#8350,.T.);
#11446=ORIENTED_EDGE('',*,*,#8347,.T.);
#11447=ORIENTED_EDGE('',*,*,#8344,.T.);
#11448=ORIENTED_EDGE('',*,*,#8341,.T.);
#11449=ORIENTED_EDGE('',*,*,#8338,.T.);
#11450=ORIENTED_EDGE('',*,*,#8335,.T.);
#11451=ORIENTED_EDGE('',*,*,#8332,.T.);
#11452=ORIENTED_EDGE('',*,*,#8329,.T.);
#11453=ORIENTED_EDGE('',*,*,#8326,.T.);
#11454=ORIENTED_EDGE('',*,*,#8323,.T.);
#11455=ORIENTED_EDGE('',*,*,#8320,.T.);
#11456=ORIENTED_EDGE('',*,*,#8317,.T.);
#11457=ORIENTED_EDGE('',*,*,#8314,.T.);
#11458=ORIENTED_EDGE('',*,*,#8311,.T.);
#11459=ORIENTED_EDGE('',*,*,#8308,.T.);
#11460=ORIENTED_EDGE('',*,*,#8305,.T.);
#11461=ORIENTED_EDGE('',*,*,#8302,.T.);
#11462=ORIENTED_EDGE('',*,*,#8299,.T.);
#11463=ORIENTED_EDGE('',*,*,#8296,.T.);
#11464=ORIENTED_EDGE('',*,*,#8293,.T.);
#11465=ORIENTED_EDGE('',*,*,#8290,.T.);
#11466=ORIENTED_EDGE('',*,*,#8287,.T.);
#11467=ORIENTED_EDGE('',*,*,#8284,.T.);
#11468=ORIENTED_EDGE('',*,*,#8281,.T.);
#11469=ORIENTED_EDGE('',*,*,#8278,.T.);
#11470=ORIENTED_EDGE('',*,*,#8275,.T.);
#11471=ORIENTED_EDGE('',*,*,#8272,.T.);
#11472=ORIENTED_EDGE('',*,*,#8269,.T.);
#11473=ORIENTED_EDGE('',*,*,#8266,.T.);
#11474=ORIENTED_EDGE('',*,*,#8263,.T.);
#11475=ORIENTED_EDGE('',*,*,#8260,.T.);
#11476=ORIENTED_EDGE('',*,*,#8257,.T.);
#11477=ORIENTED_EDGE('',*,*,#8254,.T.);
#11478=ORIENTED_EDGE('',*,*,#8251,.T.);
#11479=ORIENTED_EDGE('',*,*,#8248,.T.);
#11480=ORIENTED_EDGE('',*,*,#8245,.T.);
#11481=ORIENTED_EDGE('',*,*,#8242,.T.);
#11482=ORIENTED_EDGE('',*,*,#8239,.T.);
#11483=ORIENTED_EDGE('',*,*,#8236,.T.);
#11484=ORIENTED_EDGE('',*,*,#8616,.T.);
#11485=ORIENTED_EDGE('',*,*,#8234,.T.);
#11486=ORIENTED_EDGE('',*,*,#8238,.T.);
#11487=ORIENTED_EDGE('',*,*,#8241,.T.);
#11488=ORIENTED_EDGE('',*,*,#8244,.T.);
#11489=ORIENTED_EDGE('',*,*,#8247,.T.);
#11490=ORIENTED_EDGE('',*,*,#8250,.T.);
#11491=ORIENTED_EDGE('',*,*,#8253,.T.);
#11492=ORIENTED_EDGE('',*,*,#8256,.T.);
#11493=ORIENTED_EDGE('',*,*,#8259,.T.);
#11494=ORIENTED_EDGE('',*,*,#8262,.T.);
#11495=ORIENTED_EDGE('',*,*,#8265,.T.);
#11496=ORIENTED_EDGE('',*,*,#8268,.T.);
#11497=ORIENTED_EDGE('',*,*,#8271,.T.);
#11498=ORIENTED_EDGE('',*,*,#8274,.T.);
#11499=ORIENTED_EDGE('',*,*,#8277,.T.);
#11500=ORIENTED_EDGE('',*,*,#8280,.T.);
#11501=ORIENTED_EDGE('',*,*,#8283,.T.);
#11502=ORIENTED_EDGE('',*,*,#8286,.T.);
#11503=ORIENTED_EDGE('',*,*,#8289,.T.);
#11504=ORIENTED_EDGE('',*,*,#8292,.T.);
#11505=ORIENTED_EDGE('',*,*,#8295,.T.);
#11506=ORIENTED_EDGE('',*,*,#8298,.T.);
#11507=ORIENTED_EDGE('',*,*,#8301,.T.);
#11508=ORIENTED_EDGE('',*,*,#8304,.T.);
#11509=ORIENTED_EDGE('',*,*,#8307,.T.);
#11510=ORIENTED_EDGE('',*,*,#8310,.T.);
#11511=ORIENTED_EDGE('',*,*,#8313,.T.);
#11512=ORIENTED_EDGE('',*,*,#8316,.T.);
#11513=ORIENTED_EDGE('',*,*,#8319,.T.);
#11514=ORIENTED_EDGE('',*,*,#8322,.T.);
#11515=ORIENTED_EDGE('',*,*,#8325,.T.);
#11516=ORIENTED_EDGE('',*,*,#8328,.T.);
#11517=ORIENTED_EDGE('',*,*,#8331,.T.);
#11518=ORIENTED_EDGE('',*,*,#8334,.T.);
#11519=ORIENTED_EDGE('',*,*,#8337,.T.);
#11520=ORIENTED_EDGE('',*,*,#8340,.T.);
#11521=ORIENTED_EDGE('',*,*,#8343,.T.);
#11522=ORIENTED_EDGE('',*,*,#8346,.T.);
#11523=ORIENTED_EDGE('',*,*,#8349,.T.);
#11524=ORIENTED_EDGE('',*,*,#8352,.T.);
#11525=ORIENTED_EDGE('',*,*,#8355,.T.);
#11526=ORIENTED_EDGE('',*,*,#8358,.T.);
#11527=ORIENTED_EDGE('',*,*,#8361,.T.);
#11528=ORIENTED_EDGE('',*,*,#8364,.T.);
#11529=ORIENTED_EDGE('',*,*,#8367,.T.);
#11530=ORIENTED_EDGE('',*,*,#8370,.T.);
#11531=ORIENTED_EDGE('',*,*,#8373,.T.);
#11532=ORIENTED_EDGE('',*,*,#8376,.T.);
#11533=ORIENTED_EDGE('',*,*,#8379,.T.);
#11534=ORIENTED_EDGE('',*,*,#8382,.T.);
#11535=ORIENTED_EDGE('',*,*,#8385,.T.);
#11536=ORIENTED_EDGE('',*,*,#8388,.T.);
#11537=ORIENTED_EDGE('',*,*,#8391,.T.);
#11538=ORIENTED_EDGE('',*,*,#8394,.T.);
#11539=ORIENTED_EDGE('',*,*,#8397,.T.);
#11540=ORIENTED_EDGE('',*,*,#8400,.T.);
#11541=ORIENTED_EDGE('',*,*,#8403,.T.);
#11542=ORIENTED_EDGE('',*,*,#8406,.T.);
#11543=ORIENTED_EDGE('',*,*,#8409,.T.);
#11544=ORIENTED_EDGE('',*,*,#8412,.T.);
#11545=ORIENTED_EDGE('',*,*,#8415,.T.);
#11546=ORIENTED_EDGE('',*,*,#8418,.T.);
#11547=ORIENTED_EDGE('',*,*,#8421,.T.);
#11548=ORIENTED_EDGE('',*,*,#8424,.T.);
#11549=ORIENTED_EDGE('',*,*,#8427,.T.);
#11550=ORIENTED_EDGE('',*,*,#8430,.T.);
#11551=ORIENTED_EDGE('',*,*,#8433,.T.);
#11552=ORIENTED_EDGE('',*,*,#8436,.T.);
#11553=ORIENTED_EDGE('',*,*,#8439,.T.);
#11554=ORIENTED_EDGE('',*,*,#8442,.T.);
#11555=ORIENTED_EDGE('',*,*,#8445,.T.);
#11556=ORIENTED_EDGE('',*,*,#8448,.T.);
#11557=ORIENTED_EDGE('',*,*,#8451,.T.);
#11558=ORIENTED_EDGE('',*,*,#8454,.T.);
#11559=ORIENTED_EDGE('',*,*,#8457,.T.);
#11560=ORIENTED_EDGE('',*,*,#8460,.T.);
#11561=ORIENTED_EDGE('',*,*,#8463,.T.);
#11562=ORIENTED_EDGE('',*,*,#8466,.T.);
#11563=ORIENTED_EDGE('',*,*,#8469,.T.);
#11564=ORIENTED_EDGE('',*,*,#8472,.T.);
#11565=ORIENTED_EDGE('',*,*,#8475,.T.);
#11566=ORIENTED_EDGE('',*,*,#8478,.T.);
#11567=ORIENTED_EDGE('',*,*,#8481,.T.);
#11568=ORIENTED_EDGE('',*,*,#8484,.T.);
#11569=ORIENTED_EDGE('',*,*,#8487,.T.);
#11570=ORIENTED_EDGE('',*,*,#8490,.T.);
#11571=ORIENTED_EDGE('',*,*,#8493,.T.);
#11572=ORIENTED_EDGE('',*,*,#8496,.T.);
#11573=ORIENTED_EDGE('',*,*,#8499,.T.);
#11574=ORIENTED_EDGE('',*,*,#8502,.T.);
#11575=ORIENTED_EDGE('',*,*,#8505,.T.);
#11576=ORIENTED_EDGE('',*,*,#8508,.T.);
#11577=ORIENTED_EDGE('',*,*,#8511,.T.);
#11578=ORIENTED_EDGE('',*,*,#8514,.T.);
#11579=ORIENTED_EDGE('',*,*,#8517,.T.);
#11580=ORIENTED_EDGE('',*,*,#8520,.T.);
#11581=ORIENTED_EDGE('',*,*,#8523,.T.);
#11582=ORIENTED_EDGE('',*,*,#8526,.T.);
#11583=ORIENTED_EDGE('',*,*,#8529,.T.);
#11584=ORIENTED_EDGE('',*,*,#8532,.T.);
#11585=ORIENTED_EDGE('',*,*,#8535,.T.);
#11586=ORIENTED_EDGE('',*,*,#8538,.T.);
#11587=ORIENTED_EDGE('',*,*,#8541,.T.);
#11588=ORIENTED_EDGE('',*,*,#8544,.T.);
#11589=ORIENTED_EDGE('',*,*,#8547,.T.);
#11590=ORIENTED_EDGE('',*,*,#8550,.T.);
#11591=ORIENTED_EDGE('',*,*,#8553,.T.);
#11592=ORIENTED_EDGE('',*,*,#8556,.T.);
#11593=ORIENTED_EDGE('',*,*,#8559,.T.);
#11594=ORIENTED_EDGE('',*,*,#8562,.T.);
#11595=ORIENTED_EDGE('',*,*,#8565,.T.);
#11596=ORIENTED_EDGE('',*,*,#8568,.T.);
#11597=ORIENTED_EDGE('',*,*,#8571,.T.);
#11598=ORIENTED_EDGE('',*,*,#8574,.T.);
#11599=ORIENTED_EDGE('',*,*,#8577,.T.);
#11600=ORIENTED_EDGE('',*,*,#8580,.T.);
#11601=ORIENTED_EDGE('',*,*,#8583,.T.);
#11602=ORIENTED_EDGE('',*,*,#8586,.T.);
#11603=ORIENTED_EDGE('',*,*,#8589,.T.);
#11604=ORIENTED_EDGE('',*,*,#8592,.T.);
#11605=ORIENTED_EDGE('',*,*,#8595,.T.);
#11606=ORIENTED_EDGE('',*,*,#8598,.T.);
#11607=ORIENTED_EDGE('',*,*,#8601,.T.);
#11608=ORIENTED_EDGE('',*,*,#8604,.T.);
#11609=ORIENTED_EDGE('',*,*,#8607,.T.);
#11610=ORIENTED_EDGE('',*,*,#8610,.T.);
#11611=ORIENTED_EDGE('',*,*,#8613,.T.);
#12950=CYLINDRICAL_SURFACE('',#14963,0.164999999999999);
#12951=CYLINDRICAL_SURFACE('',#14967,0.165);
#12952=CYLINDRICAL_SURFACE('',#14971,0.165);
#12953=CYLINDRICAL_SURFACE('',#14975,0.164999999999999);
#13354=ADVANCED_FACE('',(#1876),#12950,.F.);
#13355=ADVANCED_FACE('',(#1877),#1251,.F.);
#13356=ADVANCED_FACE('',(#1878),#12951,.F.);
#13357=ADVANCED_FACE('',(#1879),#1252,.F.);
#13358=ADVANCED_FACE('',(#1880),#12952,.F.);
#13359=ADVANCED_FACE('',(#1881),#1253,.F.);
#13360=ADVANCED_FACE('',(#1882),#12953,.F.);
#13361=ADVANCED_FACE('',(#1883),#1254,.F.);
#13362=ADVANCED_FACE('',(#1884),#1255,.T.);
#13363=ADVANCED_FACE('',(#1885,#1001,#1002,#1003,#1004),#1256,.T.);
#13364=ADVANCED_FACE('',(#1886),#1257,.T.);
#13365=ADVANCED_FACE('',(#1887),#1258,.T.);
#13366=ADVANCED_FACE('',(#1888),#1259,.T.);
#13367=ADVANCED_FACE('',(#1889),#1260,.T.);
#13368=ADVANCED_FACE('',(#1890),#1261,.T.);
#13369=ADVANCED_FACE('',(#1891),#1262,.T.);
#13370=ADVANCED_FACE('',(#1892),#1263,.T.);
#13371=ADVANCED_FACE('',(#1893),#1264,.T.);
#13372=ADVANCED_FACE('',(#1894),#1265,.T.);
#13373=ADVANCED_FACE('',(#1895),#1266,.T.);
#13374=ADVANCED_FACE('',(#1896),#1267,.T.);
#13375=ADVANCED_FACE('',(#1897),#1268,.T.);
#13376=ADVANCED_FACE('',(#1898),#1269,.T.);
#13377=ADVANCED_FACE('',(#1899),#1270,.T.);
#13378=ADVANCED_FACE('',(#1900),#1271,.T.);
#13379=ADVANCED_FACE('',(#1901),#1272,.T.);
#13380=ADVANCED_FACE('',(#1902),#1273,.T.);
#13381=ADVANCED_FACE('',(#1903),#1274,.T.);
#13382=ADVANCED_FACE('',(#1904),#1275,.T.);
#13383=ADVANCED_FACE('',(#1905),#1276,.T.);
#13384=ADVANCED_FACE('',(#1906),#1277,.T.);
#13385=ADVANCED_FACE('',(#1907),#1278,.T.);
#13386=ADVANCED_FACE('',(#1908),#1279,.T.);
#13387=ADVANCED_FACE('',(#1909),#1280,.T.);
#13388=ADVANCED_FACE('',(#1910),#1281,.T.);
#13389=ADVANCED_FACE('',(#1911),#1282,.T.);
#13390=ADVANCED_FACE('',(#1912),#1283,.T.);
#13391=ADVANCED_FACE('',(#1913),#1284,.T.);
#13392=ADVANCED_FACE('',(#1914),#1285,.T.);
#13393=ADVANCED_FACE('',(#1915),#1286,.T.);
#13394=ADVANCED_FACE('',(#1916),#1287,.T.);
#13395=ADVANCED_FACE('',(#1917),#1288,.T.);
#13396=ADVANCED_FACE('',(#1918),#1289,.T.);
#13397=ADVANCED_FACE('',(#1919),#1290,.T.);
#13398=ADVANCED_FACE('',(#1920),#1291,.T.);
#13399=ADVANCED_FACE('',(#1921),#1292,.T.);
#13400=ADVANCED_FACE('',(#1922),#1293,.T.);
#13401=ADVANCED_FACE('',(#1923),#1294,.T.);
#13402=ADVANCED_FACE('',(#1924),#1295,.T.);
#13403=ADVANCED_FACE('',(#1925),#1296,.T.);
#13404=ADVANCED_FACE('',(#1926),#1297,.T.);
#13405=ADVANCED_FACE('',(#1927),#1298,.T.);
#13406=ADVANCED_FACE('',(#1928),#1299,.T.);
#13407=ADVANCED_FACE('',(#1929),#1300,.T.);
#13408=ADVANCED_FACE('',(#1930),#1301,.T.);
#13409=ADVANCED_FACE('',(#1931),#1302,.T.);
#13410=ADVANCED_FACE('',(#1932),#1303,.T.);
#13411=ADVANCED_FACE('',(#1933),#1304,.T.);
#13412=ADVANCED_FACE('',(#1934),#1305,.T.);
#13413=ADVANCED_FACE('',(#1935),#1306,.T.);
#13414=ADVANCED_FACE('',(#1936),#1307,.T.);
#13415=ADVANCED_FACE('',(#1937),#1308,.T.);
#13416=ADVANCED_FACE('',(#1938),#1309,.T.);
#13417=ADVANCED_FACE('',(#1939),#1310,.T.);
#13418=ADVANCED_FACE('',(#1940),#1311,.T.);
#13419=ADVANCED_FACE('',(#1941),#1312,.T.);
#13420=ADVANCED_FACE('',(#1942),#1313,.T.);
#13421=ADVANCED_FACE('',(#1943),#1314,.T.);
#13422=ADVANCED_FACE('',(#1944),#1315,.T.);
#13423=ADVANCED_FACE('',(#1945),#1316,.T.);
#13424=ADVANCED_FACE('',(#1946),#1317,.T.);
#13425=ADVANCED_FACE('',(#1947),#1318,.T.);
#13426=ADVANCED_FACE('',(#1948),#1319,.T.);
#13427=ADVANCED_FACE('',(#1949),#1320,.T.);
#13428=ADVANCED_FACE('',(#1950),#1321,.T.);
#13429=ADVANCED_FACE('',(#1951),#1322,.T.);
#13430=ADVANCED_FACE('',(#1952),#1323,.T.);
#13431=ADVANCED_FACE('',(#1953),#1324,.T.);
#13432=ADVANCED_FACE('',(#1954),#1325,.T.);
#13433=ADVANCED_FACE('',(#1955),#1326,.T.);
#13434=ADVANCED_FACE('',(#1956),#1327,.T.);
#13435=ADVANCED_FACE('',(#1957),#1328,.T.);
#13436=ADVANCED_FACE('',(#1958),#1329,.T.);
#13437=ADVANCED_FACE('',(#1959),#1330,.T.);
#13438=ADVANCED_FACE('',(#1960),#1331,.T.);
#13439=ADVANCED_FACE('',(#1961),#1332,.T.);
#13440=ADVANCED_FACE('',(#1962),#1333,.T.);
#13441=ADVANCED_FACE('',(#1963),#1334,.T.);
#13442=ADVANCED_FACE('',(#1964),#1335,.T.);
#13443=ADVANCED_FACE('',(#1965),#1336,.T.);
#13444=ADVANCED_FACE('',(#1966),#1337,.T.);
#13445=ADVANCED_FACE('',(#1967),#1338,.T.);
#13446=ADVANCED_FACE('',(#1968),#1339,.T.);
#13447=ADVANCED_FACE('',(#1969),#1340,.T.);
#13448=ADVANCED_FACE('',(#1970),#1341,.T.);
#13449=ADVANCED_FACE('',(#1971),#1342,.T.);
#13450=ADVANCED_FACE('',(#1972),#1343,.T.);
#13451=ADVANCED_FACE('',(#1973),#1344,.T.);
#13452=ADVANCED_FACE('',(#1974),#1345,.T.);
#13453=ADVANCED_FACE('',(#1975),#1346,.T.);
#13454=ADVANCED_FACE('',(#1976),#1347,.T.);
#13455=ADVANCED_FACE('',(#1977),#1348,.T.);
#13456=ADVANCED_FACE('',(#1978),#1349,.T.);
#13457=ADVANCED_FACE('',(#1979),#1350,.T.);
#13458=ADVANCED_FACE('',(#1980),#1351,.T.);
#13459=ADVANCED_FACE('',(#1981),#1352,.T.);
#13460=ADVANCED_FACE('',(#1982),#1353,.T.);
#13461=ADVANCED_FACE('',(#1983),#1354,.T.);
#13462=ADVANCED_FACE('',(#1984),#1355,.T.);
#13463=ADVANCED_FACE('',(#1985),#1356,.T.);
#13464=ADVANCED_FACE('',(#1986),#1357,.T.);
#13465=ADVANCED_FACE('',(#1987),#1358,.T.);
#13466=ADVANCED_FACE('',(#1988),#1359,.T.);
#13467=ADVANCED_FACE('',(#1989),#1360,.T.);
#13468=ADVANCED_FACE('',(#1990),#1361,.T.);
#13469=ADVANCED_FACE('',(#1991),#1362,.T.);
#13470=ADVANCED_FACE('',(#1992),#1363,.T.);
#13471=ADVANCED_FACE('',(#1993),#1364,.T.);
#13472=ADVANCED_FACE('',(#1994),#1365,.T.);
#13473=ADVANCED_FACE('',(#1995),#1366,.T.);
#13474=ADVANCED_FACE('',(#1996),#1367,.T.);
#13475=ADVANCED_FACE('',(#1997),#1368,.T.);
#13476=ADVANCED_FACE('',(#1998),#1369,.T.);
#13477=ADVANCED_FACE('',(#1999),#1370,.T.);
#13478=ADVANCED_FACE('',(#2000),#1371,.T.);
#13479=ADVANCED_FACE('',(#2001),#1372,.T.);
#13480=ADVANCED_FACE('',(#2002),#1373,.T.);
#13481=ADVANCED_FACE('',(#2003),#1374,.T.);
#13482=ADVANCED_FACE('',(#2004),#1375,.T.);
#13483=ADVANCED_FACE('',(#2005),#1376,.T.);
#13484=ADVANCED_FACE('',(#2006),#1377,.T.);
#13485=ADVANCED_FACE('',(#2007),#1378,.T.);
#13486=ADVANCED_FACE('',(#2008),#1379,.T.);
#13487=ADVANCED_FACE('',(#2009),#1380,.T.);
#13488=ADVANCED_FACE('',(#2010),#1381,.T.);
#13489=ADVANCED_FACE('',(#2011),#1382,.T.);
#13490=ADVANCED_FACE('',(#2012),#1383,.T.);
#13491=ADVANCED_FACE('',(#2013),#1384,.F.);
#13787=CLOSED_SHELL('',(#13354,#13355,#13356,#13357,#13358,#13359,#13360,
#13361,#13362,#13363,#13364,#13365,#13366,#13367,#13368,#13369,#13370,#13371,
#13372,#13373,#13374,#13375,#13376,#13377,#13378,#13379,#13380,#13381,#13382,
#13383,#13384,#13385,#13386,#13387,#13388,#13389,#13390,#13391,#13392,#13393,
#13394,#13395,#13396,#13397,#13398,#13399,#13400,#13401,#13402,#13403,#13404,
#13405,#13406,#13407,#13408,#13409,#13410,#13411,#13412,#13413,#13414,#13415,
#13416,#13417,#13418,#13419,#13420,#13421,#13422,#13423,#13424,#13425,#13426,
#13427,#13428,#13429,#13430,#13431,#13432,#13433,#13434,#13435,#13436,#13437,
#13438,#13439,#13440,#13441,#13442,#13443,#13444,#13445,#13446,#13447,#13448,
#13449,#13450,#13451,#13452,#13453,#13454,#13455,#13456,#13457,#13458,#13459,
#13460,#13461,#13462,#13463,#13464,#13465,#13466,#13467,#13468,#13469,#13470,
#13471,#13472,#13473,#13474,#13475,#13476,#13477,#13478,#13479,#13480,#13481,
#13482,#13483,#13484,#13485,#13486,#13487,#13488,#13489,#13490,#13491));
#14962=AXIS2_PLACEMENT_3D('',#21454,#17400,#17401);
#14963=AXIS2_PLACEMENT_3D('',#21455,#17402,#17403);
#14964=AXIS2_PLACEMENT_3D('',#21457,#17404,#17405);
#14965=AXIS2_PLACEMENT_3D('',#21460,#17407,#17408);
#14966=AXIS2_PLACEMENT_3D('',#21461,#17409,#17410);
#14967=AXIS2_PLACEMENT_3D('',#21462,#17411,#17412);
#14968=AXIS2_PLACEMENT_3D('',#21464,#17413,#17414);
#14969=AXIS2_PLACEMENT_3D('',#21467,#17416,#17417);
#14970=AXIS2_PLACEMENT_3D('',#21468,#17418,#17419);
#14971=AXIS2_PLACEMENT_3D('',#21469,#17420,#17421);
#14972=AXIS2_PLACEMENT_3D('',#21471,#17422,#17423);
#14973=AXIS2_PLACEMENT_3D('',#21474,#17425,#17426);
#14974=AXIS2_PLACEMENT_3D('',#21475,#17427,#17428);
#14975=AXIS2_PLACEMENT_3D('',#21476,#17429,#17430);
#14976=AXIS2_PLACEMENT_3D('',#21478,#17431,#17432);
#14977=AXIS2_PLACEMENT_3D('',#21481,#17434,#17435);
#14978=AXIS2_PLACEMENT_3D('',#21482,#17436,#17437);
#14979=AXIS2_PLACEMENT_3D('',#21483,#17438,#17439);
#14980=AXIS2_PLACEMENT_3D('',#21492,#17444,#17445);
#14981=AXIS2_PLACEMENT_3D('',#21498,#17449,#17450);
#14982=AXIS2_PLACEMENT_3D('',#21504,#17454,#17455);
#14983=AXIS2_PLACEMENT_3D('',#21510,#17459,#17460);
#14984=AXIS2_PLACEMENT_3D('',#21516,#17464,#17465);
#14985=AXIS2_PLACEMENT_3D('',#21522,#17469,#17470);
#14986=AXIS2_PLACEMENT_3D('',#21528,#17474,#17475);
#14987=AXIS2_PLACEMENT_3D('',#21534,#17479,#17480);
#14988=AXIS2_PLACEMENT_3D('',#21540,#17484,#17485);
#14989=AXIS2_PLACEMENT_3D('',#21546,#17489,#17490);
#14990=AXIS2_PLACEMENT_3D('',#21552,#17494,#17495);
#14991=AXIS2_PLACEMENT_3D('',#21558,#17499,#17500);
#14992=AXIS2_PLACEMENT_3D('',#21564,#17504,#17505);
#14993=AXIS2_PLACEMENT_3D('',#21570,#17509,#17510);
#14994=AXIS2_PLACEMENT_3D('',#21576,#17514,#17515);
#14995=AXIS2_PLACEMENT_3D('',#21582,#17519,#17520);
#14996=AXIS2_PLACEMENT_3D('',#21588,#17524,#17525);
#14997=AXIS2_PLACEMENT_3D('',#21594,#17529,#17530);
#14998=AXIS2_PLACEMENT_3D('',#21600,#17534,#17535);
#14999=AXIS2_PLACEMENT_3D('',#21606,#17539,#17540);
#15000=AXIS2_PLACEMENT_3D('',#21612,#17544,#17545);
#15001=AXIS2_PLACEMENT_3D('',#21618,#17549,#17550);
#15002=AXIS2_PLACEMENT_3D('',#21624,#17554,#17555);
#15003=AXIS2_PLACEMENT_3D('',#21630,#17559,#17560);
#15004=AXIS2_PLACEMENT_3D('',#21636,#17564,#17565);
#15005=AXIS2_PLACEMENT_3D('',#21642,#17569,#17570);
#15006=AXIS2_PLACEMENT_3D('',#21648,#17574,#17575);
#15007=AXIS2_PLACEMENT_3D('',#21654,#17579,#17580);
#15008=AXIS2_PLACEMENT_3D('',#21660,#17584,#17585);
#15009=AXIS2_PLACEMENT_3D('',#21666,#17589,#17590);
#15010=AXIS2_PLACEMENT_3D('',#21672,#17594,#17595);
#15011=AXIS2_PLACEMENT_3D('',#21678,#17599,#17600);
#15012=AXIS2_PLACEMENT_3D('',#21684,#17604,#17605);
#15013=AXIS2_PLACEMENT_3D('',#21690,#17609,#17610);
#15014=AXIS2_PLACEMENT_3D('',#21696,#17614,#17615);
#15015=AXIS2_PLACEMENT_3D('',#21702,#17619,#17620);
#15016=AXIS2_PLACEMENT_3D('',#21708,#17624,#17625);
#15017=AXIS2_PLACEMENT_3D('',#21714,#17629,#17630);
#15018=AXIS2_PLACEMENT_3D('',#21720,#17634,#17635);
#15019=AXIS2_PLACEMENT_3D('',#21726,#17639,#17640);
#15020=AXIS2_PLACEMENT_3D('',#21732,#17644,#17645);
#15021=AXIS2_PLACEMENT_3D('',#21738,#17649,#17650);
#15022=AXIS2_PLACEMENT_3D('',#21744,#17654,#17655);
#15023=AXIS2_PLACEMENT_3D('',#21750,#17659,#17660);
#15024=AXIS2_PLACEMENT_3D('',#21756,#17664,#17665);
#15025=AXIS2_PLACEMENT_3D('',#21762,#17669,#17670);
#15026=AXIS2_PLACEMENT_3D('',#21768,#17674,#17675);
#15027=AXIS2_PLACEMENT_3D('',#21774,#17679,#17680);
#15028=AXIS2_PLACEMENT_3D('',#21780,#17684,#17685);
#15029=AXIS2_PLACEMENT_3D('',#21786,#17689,#17690);
#15030=AXIS2_PLACEMENT_3D('',#21792,#17694,#17695);
#15031=AXIS2_PLACEMENT_3D('',#21798,#17699,#17700);
#15032=AXIS2_PLACEMENT_3D('',#21804,#17704,#17705);
#15033=AXIS2_PLACEMENT_3D('',#21810,#17709,#17710);
#15034=AXIS2_PLACEMENT_3D('',#21816,#17714,#17715);
#15035=AXIS2_PLACEMENT_3D('',#21822,#17719,#17720);
#15036=AXIS2_PLACEMENT_3D('',#21828,#17724,#17725);
#15037=AXIS2_PLACEMENT_3D('',#21834,#17729,#17730);
#15038=AXIS2_PLACEMENT_3D('',#21840,#17734,#17735);
#15039=AXIS2_PLACEMENT_3D('',#21846,#17739,#17740);
#15040=AXIS2_PLACEMENT_3D('',#21852,#17744,#17745);
#15041=AXIS2_PLACEMENT_3D('',#21858,#17749,#17750);
#15042=AXIS2_PLACEMENT_3D('',#21864,#17754,#17755);
#15043=AXIS2_PLACEMENT_3D('',#21870,#17759,#17760);
#15044=AXIS2_PLACEMENT_3D('',#21876,#17764,#17765);
#15045=AXIS2_PLACEMENT_3D('',#21882,#17769,#17770);
#15046=AXIS2_PLACEMENT_3D('',#21888,#17774,#17775);
#15047=AXIS2_PLACEMENT_3D('',#21894,#17779,#17780);
#15048=AXIS2_PLACEMENT_3D('',#21900,#17784,#17785);
#15049=AXIS2_PLACEMENT_3D('',#21906,#17789,#17790);
#15050=AXIS2_PLACEMENT_3D('',#21912,#17794,#17795);
#15051=AXIS2_PLACEMENT_3D('',#21918,#17799,#17800);
#15052=AXIS2_PLACEMENT_3D('',#21924,#17804,#17805);
#15053=AXIS2_PLACEMENT_3D('',#21930,#17809,#17810);
#15054=AXIS2_PLACEMENT_3D('',#21936,#17814,#17815);
#15055=AXIS2_PLACEMENT_3D('',#21942,#17819,#17820);
#15056=AXIS2_PLACEMENT_3D('',#21948,#17824,#17825);
#15057=AXIS2_PLACEMENT_3D('',#21954,#17829,#17830);
#15058=AXIS2_PLACEMENT_3D('',#21960,#17834,#17835);
#15059=AXIS2_PLACEMENT_3D('',#21966,#17839,#17840);
#15060=AXIS2_PLACEMENT_3D('',#21972,#17844,#17845);
#15061=AXIS2_PLACEMENT_3D('',#21978,#17849,#17850);
#15062=AXIS2_PLACEMENT_3D('',#21984,#17854,#17855);
#15063=AXIS2_PLACEMENT_3D('',#21990,#17859,#17860);
#15064=AXIS2_PLACEMENT_3D('',#21996,#17864,#17865);
#15065=AXIS2_PLACEMENT_3D('',#22002,#17869,#17870);
#15066=AXIS2_PLACEMENT_3D('',#22008,#17874,#17875);
#15067=AXIS2_PLACEMENT_3D('',#22014,#17879,#17880);
#15068=AXIS2_PLACEMENT_3D('',#22020,#17884,#17885);
#15069=AXIS2_PLACEMENT_3D('',#22026,#17889,#17890);
#15070=AXIS2_PLACEMENT_3D('',#22032,#17894,#17895);
#15071=AXIS2_PLACEMENT_3D('',#22038,#17899,#17900);
#15072=AXIS2_PLACEMENT_3D('',#22044,#17904,#17905);
#15073=AXIS2_PLACEMENT_3D('',#22050,#17909,#17910);
#15074=AXIS2_PLACEMENT_3D('',#22056,#17914,#17915);
#15075=AXIS2_PLACEMENT_3D('',#22062,#17919,#17920);
#15076=AXIS2_PLACEMENT_3D('',#22068,#17924,#17925);
#15077=AXIS2_PLACEMENT_3D('',#22074,#17929,#17930);
#15078=AXIS2_PLACEMENT_3D('',#22080,#17934,#17935);
#15079=AXIS2_PLACEMENT_3D('',#22086,#17939,#17940);
#15080=AXIS2_PLACEMENT_3D('',#22092,#17944,#17945);
#15081=AXIS2_PLACEMENT_3D('',#22098,#17949,#17950);
#15082=AXIS2_PLACEMENT_3D('',#22104,#17954,#17955);
#15083=AXIS2_PLACEMENT_3D('',#22110,#17959,#17960);
#15084=AXIS2_PLACEMENT_3D('',#22116,#17964,#17965);
#15085=AXIS2_PLACEMENT_3D('',#22122,#17969,#17970);
#15086=AXIS2_PLACEMENT_3D('',#22128,#17974,#17975);
#15087=AXIS2_PLACEMENT_3D('',#22134,#17979,#17980);
#15088=AXIS2_PLACEMENT_3D('',#22140,#17984,#17985);
#15089=AXIS2_PLACEMENT_3D('',#22146,#17989,#17990);
#15090=AXIS2_PLACEMENT_3D('',#22152,#17994,#17995);
#15091=AXIS2_PLACEMENT_3D('',#22158,#17999,#18000);
#15092=AXIS2_PLACEMENT_3D('',#22164,#18004,#18005);
#15093=AXIS2_PLACEMENT_3D('',#22170,#18009,#18010);
#15094=AXIS2_PLACEMENT_3D('',#22176,#18014,#18015);
#15095=AXIS2_PLACEMENT_3D('',#22182,#18019,#18020);
#15096=AXIS2_PLACEMENT_3D('',#22188,#18024,#18025);
#15097=AXIS2_PLACEMENT_3D('',#22194,#18029,#18030);
#15098=AXIS2_PLACEMENT_3D('',#22200,#18034,#18035);
#15099=AXIS2_PLACEMENT_3D('',#22206,#18039,#18040);
#15100=AXIS2_PLACEMENT_3D('',#22212,#18044,#18045);
#15101=AXIS2_PLACEMENT_3D('',#22218,#18049,#18050);
#15102=AXIS2_PLACEMENT_3D('',#22224,#18054,#18055);
#15103=AXIS2_PLACEMENT_3D('',#22230,#18059,#18060);
#15104=AXIS2_PLACEMENT_3D('',#22236,#18064,#18065);
#15105=AXIS2_PLACEMENT_3D('',#22242,#18069,#18070);
#15106=AXIS2_PLACEMENT_3D('',#22248,#18074,#18075);
#15107=AXIS2_PLACEMENT_3D('',#22251,#18078,#18079);
#15108=AXIS2_PLACEMENT_3D('',#22252,#18080,#18081);
#17400=DIRECTION('axis',(0.,0.,1.));
#17401=DIRECTION('refdir',(1.,0.,0.));
#17402=DIRECTION('center_axis',(0.,0.,1.));
#17403=DIRECTION('ref_axis',(1.,0.,0.));
#17404=DIRECTION('center_axis',(0.,0.,1.));
#17405=DIRECTION('ref_axis',(1.,0.,0.));
#17406=DIRECTION('',(0.,0.,1.));
#17407=DIRECTION('center_axis',(0.,0.,1.));
#17408=DIRECTION('ref_axis',(1.,0.,0.));
#17409=DIRECTION('center_axis',(0.,0.,1.));
#17410=DIRECTION('ref_axis',(1.,0.,0.));
#17411=DIRECTION('center_axis',(0.,0.,1.));
#17412=DIRECTION('ref_axis',(1.,0.,0.));
#17413=DIRECTION('center_axis',(0.,0.,1.));
#17414=DIRECTION('ref_axis',(1.,0.,0.));
#17415=DIRECTION('',(0.,0.,1.));
#17416=DIRECTION('center_axis',(0.,0.,1.));
#17417=DIRECTION('ref_axis',(1.,0.,0.));
#17418=DIRECTION('center_axis',(0.,0.,1.));
#17419=DIRECTION('ref_axis',(1.,0.,0.));
#17420=DIRECTION('center_axis',(0.,0.,1.));
#17421=DIRECTION('ref_axis',(1.,0.,0.));
#17422=DIRECTION('center_axis',(0.,0.,1.));
#17423=DIRECTION('ref_axis',(1.,0.,0.));
#17424=DIRECTION('',(0.,0.,1.));
#17425=DIRECTION('center_axis',(0.,0.,1.));
#17426=DIRECTION('ref_axis',(1.,0.,0.));
#17427=DIRECTION('center_axis',(0.,0.,1.));
#17428=DIRECTION('ref_axis',(1.,0.,0.));
#17429=DIRECTION('center_axis',(0.,0.,1.));
#17430=DIRECTION('ref_axis',(1.,0.,0.));
#17431=DIRECTION('center_axis',(0.,0.,1.));
#17432=DIRECTION('ref_axis',(1.,0.,0.));
#17433=DIRECTION('',(0.,0.,1.));
#17434=DIRECTION('center_axis',(0.,0.,1.));
#17435=DIRECTION('ref_axis',(1.,0.,0.));
#17436=DIRECTION('center_axis',(0.,0.,1.));
#17437=DIRECTION('ref_axis',(1.,0.,0.));
#17438=DIRECTION('center_axis',(-1.,0.,0.));
#17439=DIRECTION('ref_axis',(0.,0.,1.));
#17440=DIRECTION('',(0.,0.,-1.));
#17441=DIRECTION('',(0.,1.,0.));
#17442=DIRECTION('',(0.,0.,1.));
#17443=DIRECTION('',(0.,1.,0.));
#17444=DIRECTION('center_axis',(0.,0.,-1.));
#17445=DIRECTION('ref_axis',(-1.,0.,0.));
#17446=DIRECTION('',(1.,0.,0.));
#17447=DIRECTION('',(-1.,0.,0.));
#17448=DIRECTION('',(0.,1.,0.));
#17449=DIRECTION('center_axis',(1.,0.,0.));
#17450=DIRECTION('ref_axis',(0.,0.,-1.));
#17451=DIRECTION('',(0.,0.,1.));
#17452=DIRECTION('',(0.,0.,-1.));
#17453=DIRECTION('',(0.,1.,0.));
#17454=DIRECTION('center_axis',(0.,0.,1.));
#17455=DIRECTION('ref_axis',(1.,0.,0.));
#17456=DIRECTION('',(-1.,0.,0.));
#17457=DIRECTION('',(1.,0.,0.));
#17458=DIRECTION('',(0.,1.,0.));
#17459=DIRECTION('center_axis',(0.939692620785911,0.,0.342020143325662));
#17460=DIRECTION('ref_axis',(0.342020143325662,0.,-0.939692620785911));
#17461=DIRECTION('',(-0.342020143325662,0.,0.939692620785911));
#17462=DIRECTION('',(0.342020143325662,0.,-0.939692620785911));
#17463=DIRECTION('',(0.,1.,0.));
#17464=DIRECTION('center_axis',(0.,0.,1.));
#17465=DIRECTION('ref_axis',(1.,0.,0.));
#17466=DIRECTION('',(-1.,0.,0.));
#17467=DIRECTION('',(1.,0.,0.));
#17468=DIRECTION('',(0.,1.,0.));
#17469=DIRECTION('center_axis',(-0.939692620785908,0.,0.342020143325669));
#17470=DIRECTION('ref_axis',(0.342020143325669,0.,0.939692620785908));
#17471=DIRECTION('',(-0.342020143325669,0.,-0.939692620785908));
#17472=DIRECTION('',(0.342020143325669,0.,0.939692620785908));
#17473=DIRECTION('',(0.,1.,0.));
#17474=DIRECTION('center_axis',(0.,0.,1.));
#17475=DIRECTION('ref_axis',(1.,0.,0.));
#17476=DIRECTION('',(-1.,0.,0.));
#17477=DIRECTION('',(1.,0.,0.));
#17478=DIRECTION('',(0.,1.,0.));
#17479=DIRECTION('center_axis',(0.939692620785908,0.,0.342020143325669));
#17480=DIRECTION('ref_axis',(0.342020143325669,0.,-0.939692620785908));
#17481=DIRECTION('',(-0.342020143325669,0.,0.939692620785908));
#17482=DIRECTION('',(0.342020143325669,0.,-0.939692620785908));
#17483=DIRECTION('',(0.,1.,0.));
#17484=DIRECTION('center_axis',(0.,0.,1.));
#17485=DIRECTION('ref_axis',(1.,0.,0.));
#17486=DIRECTION('',(-1.,0.,0.));
#17487=DIRECTION('',(1.,0.,0.));
#17488=DIRECTION('',(0.,1.,0.));
#17489=DIRECTION('center_axis',(-0.939692620785908,0.,0.342020143325669));
#17490=DIRECTION('ref_axis',(0.342020143325669,0.,0.939692620785908));
#17491=DIRECTION('',(-0.342020143325669,0.,-0.939692620785908));
#17492=DIRECTION('',(0.342020143325669,0.,0.939692620785908));
#17493=DIRECTION('',(0.,1.,0.));
#17494=DIRECTION('center_axis',(0.,0.,1.));
#17495=DIRECTION('ref_axis',(1.,0.,0.));
#17496=DIRECTION('',(-1.,0.,0.));
#17497=DIRECTION('',(1.,0.,0.));
#17498=DIRECTION('',(0.,1.,0.));
#17499=DIRECTION('center_axis',(0.939692620785908,0.,0.342020143325669));
#17500=DIRECTION('ref_axis',(0.342020143325669,0.,-0.939692620785908));
#17501=DIRECTION('',(-0.342020143325669,0.,0.939692620785908));
#17502=DIRECTION('',(0.342020143325669,0.,-0.939692620785908));
#17503=DIRECTION('',(0.,1.,0.));
#17504=DIRECTION('center_axis',(0.,0.,1.));
#17505=DIRECTION('ref_axis',(1.,0.,0.));
#17506=DIRECTION('',(-1.,0.,0.));
#17507=DIRECTION('',(1.,0.,0.));
#17508=DIRECTION('',(0.,1.,0.));
#17509=DIRECTION('center_axis',(-0.939692620785908,0.,0.342020143325669));
#17510=DIRECTION('ref_axis',(0.342020143325669,0.,0.939692620785908));
#17511=DIRECTION('',(-0.342020143325669,0.,-0.939692620785908));
#17512=DIRECTION('',(0.342020143325669,0.,0.939692620785908));
#17513=DIRECTION('',(0.,1.,0.));
#17514=DIRECTION('center_axis',(0.,0.,1.));
#17515=DIRECTION('ref_axis',(1.,0.,0.));
#17516=DIRECTION('',(-1.,0.,0.));
#17517=DIRECTION('',(1.,0.,0.));
#17518=DIRECTION('',(0.,1.,0.));
#17519=DIRECTION('center_axis',(0.939692620785908,0.,0.342020143325669));
#17520=DIRECTION('ref_axis',(0.342020143325669,0.,-0.939692620785908));
#17521=DIRECTION('',(-0.342020143325669,0.,0.939692620785908));
#17522=DIRECTION('',(0.342020143325669,0.,-0.939692620785908));
#17523=DIRECTION('',(0.,1.,0.));
#17524=DIRECTION('center_axis',(0.,0.,1.));
#17525=DIRECTION('ref_axis',(1.,0.,0.));
#17526=DIRECTION('',(-1.,0.,0.));
#17527=DIRECTION('',(1.,0.,0.));
#17528=DIRECTION('',(0.,1.,0.));
#17529=DIRECTION('center_axis',(-0.939692620785908,0.,0.342020143325669));
#17530=DIRECTION('ref_axis',(0.342020143325669,0.,0.939692620785908));
#17531=DIRECTION('',(-0.342020143325669,0.,-0.939692620785908));
#17532=DIRECTION('',(0.342020143325669,0.,0.939692620785908));
#17533=DIRECTION('',(0.,1.,0.));
#17534=DIRECTION('center_axis',(0.,0.,1.));
#17535=DIRECTION('ref_axis',(1.,0.,0.));
#17536=DIRECTION('',(-1.,0.,0.));
#17537=DIRECTION('',(1.,0.,0.));
#17538=DIRECTION('',(0.,1.,0.));
#17539=DIRECTION('center_axis',(0.939692620785908,0.,0.342020143325669));
#17540=DIRECTION('ref_axis',(0.342020143325669,0.,-0.939692620785908));
#17541=DIRECTION('',(-0.342020143325669,0.,0.939692620785908));
#17542=DIRECTION('',(0.342020143325669,0.,-0.939692620785908));
#17543=DIRECTION('',(0.,1.,0.));
#17544=DIRECTION('center_axis',(0.,0.,1.));
#17545=DIRECTION('ref_axis',(1.,0.,0.));
#17546=DIRECTION('',(-1.,0.,0.));
#17547=DIRECTION('',(1.,0.,0.));
#17548=DIRECTION('',(0.,1.,0.));
#17549=DIRECTION('center_axis',(-0.939692620785908,0.,0.342020143325669));
#17550=DIRECTION('ref_axis',(0.342020143325669,0.,0.939692620785908));
#17551=DIRECTION('',(-0.342020143325669,0.,-0.939692620785908));
#17552=DIRECTION('',(0.342020143325669,0.,0.939692620785908));
#17553=DIRECTION('',(0.,1.,0.));
#17554=DIRECTION('center_axis',(0.,0.,1.));
#17555=DIRECTION('ref_axis',(1.,0.,0.));
#17556=DIRECTION('',(-1.,0.,0.));
#17557=DIRECTION('',(1.,0.,0.));
#17558=DIRECTION('',(0.,1.,0.));
#17559=DIRECTION('center_axis',(0.939692620785908,0.,0.342020143325669));
#17560=DIRECTION('ref_axis',(0.342020143325669,0.,-0.939692620785908));
#17561=DIRECTION('',(-0.342020143325669,0.,0.939692620785908));
#17562=DIRECTION('',(0.342020143325669,0.,-0.939692620785908));
#17563=DIRECTION('',(0.,1.,0.));
#17564=DIRECTION('center_axis',(0.,0.,1.));
#17565=DIRECTION('ref_axis',(1.,0.,0.));
#17566=DIRECTION('',(-1.,0.,0.));
#17567=DIRECTION('',(1.,0.,0.));
#17568=DIRECTION('',(0.,1.,0.));
#17569=DIRECTION('center_axis',(-0.939692620785908,0.,0.342020143325669));
#17570=DIRECTION('ref_axis',(0.342020143325669,0.,0.939692620785908));
#17571=DIRECTION('',(-0.342020143325669,0.,-0.939692620785908));
#17572=DIRECTION('',(0.342020143325669,0.,0.939692620785908));
#17573=DIRECTION('',(0.,1.,0.));
#17574=DIRECTION('center_axis',(0.,0.,1.));
#17575=DIRECTION('ref_axis',(1.,0.,0.));
#17576=DIRECTION('',(-1.,0.,0.));
#17577=DIRECTION('',(1.,0.,0.));
#17578=DIRECTION('',(0.,1.,0.));
#17579=DIRECTION('center_axis',(0.939692620785908,0.,0.342020143325669));
#17580=DIRECTION('ref_axis',(0.342020143325669,0.,-0.939692620785908));
#17581=DIRECTION('',(-0.342020143325669,0.,0.939692620785908));
#17582=DIRECTION('',(0.342020143325669,0.,-0.939692620785908));
#17583=DIRECTION('',(0.,1.,0.));
#17584=DIRECTION('center_axis',(0.,0.,1.));
#17585=DIRECTION('ref_axis',(1.,0.,0.));
#17586=DIRECTION('',(-1.,0.,0.));
#17587=DIRECTION('',(1.,0.,0.));
#17588=DIRECTION('',(0.,1.,0.));
#17589=DIRECTION('center_axis',(-0.939692620785908,0.,0.342020143325669));
#17590=DIRECTION('ref_axis',(0.342020143325669,0.,0.939692620785908));
#17591=DIRECTION('',(-0.342020143325669,0.,-0.939692620785908));
#17592=DIRECTION('',(0.342020143325669,0.,0.939692620785908));
#17593=DIRECTION('',(0.,1.,0.));
#17594=DIRECTION('center_axis',(0.,0.,1.));
#17595=DIRECTION('ref_axis',(1.,0.,0.));
#17596=DIRECTION('',(-1.,0.,0.));
#17597=DIRECTION('',(1.,0.,0.));
#17598=DIRECTION('',(0.,1.,0.));
#17599=DIRECTION('center_axis',(0.939692620785908,0.,0.342020143325669));
#17600=DIRECTION('ref_axis',(0.342020143325669,0.,-0.939692620785908));
#17601=DIRECTION('',(-0.342020143325669,0.,0.939692620785908));
#17602=DIRECTION('',(0.342020143325669,0.,-0.939692620785908));
#17603=DIRECTION('',(0.,1.,0.));
#17604=DIRECTION('center_axis',(0.,0.,1.));
#17605=DIRECTION('ref_axis',(1.,0.,0.));
#17606=DIRECTION('',(-1.,0.,0.));
#17607=DIRECTION('',(1.,0.,0.));
#17608=DIRECTION('',(0.,1.,0.));
#17609=DIRECTION('center_axis',(-0.939692620785911,0.,0.342020143325662));
#17610=DIRECTION('ref_axis',(0.342020143325662,0.,0.939692620785911));
#17611=DIRECTION('',(-0.342020143325662,0.,-0.939692620785911));
#17612=DIRECTION('',(0.342020143325662,0.,0.939692620785911));
#17613=DIRECTION('',(0.,1.,0.));
#17614=DIRECTION('center_axis',(0.,0.,1.));
#17615=DIRECTION('ref_axis',(1.,0.,0.));
#17616=DIRECTION('',(-1.,0.,0.));
#17617=DIRECTION('',(1.,0.,0.));
#17618=DIRECTION('',(0.,1.,0.));
#17619=DIRECTION('center_axis',(0.939692620785908,0.,0.342020143325669));
#17620=DIRECTION('ref_axis',(0.342020143325669,0.,-0.939692620785908));
#17621=DIRECTION('',(-0.342020143325669,0.,0.939692620785908));
#17622=DIRECTION('',(0.342020143325669,0.,-0.939692620785908));
#17623=DIRECTION('',(0.,1.,0.));
#17624=DIRECTION('center_axis',(0.,0.,1.));
#17625=DIRECTION('ref_axis',(1.,0.,0.));
#17626=DIRECTION('',(-1.,0.,0.));
#17627=DIRECTION('',(1.,0.,0.));
#17628=DIRECTION('',(0.,1.,0.));
#17629=DIRECTION('center_axis',(-0.939692620785908,0.,0.342020143325669));
#17630=DIRECTION('ref_axis',(0.342020143325669,0.,0.939692620785908));
#17631=DIRECTION('',(-0.342020143325669,0.,-0.939692620785908));
#17632=DIRECTION('',(0.342020143325669,0.,0.939692620785908));
#17633=DIRECTION('',(0.,1.,0.));
#17634=DIRECTION('center_axis',(0.,0.,1.));
#17635=DIRECTION('ref_axis',(1.,0.,0.));
#17636=DIRECTION('',(-1.,0.,0.));
#17637=DIRECTION('',(1.,0.,0.));
#17638=DIRECTION('',(0.,1.,0.));
#17639=DIRECTION('center_axis',(0.93969262078591,0.,0.342020143325665));
#17640=DIRECTION('ref_axis',(0.342020143325665,0.,-0.93969262078591));
#17641=DIRECTION('',(-0.342020143325665,0.,0.93969262078591));
#17642=DIRECTION('',(0.342020143325665,0.,-0.93969262078591));
#17643=DIRECTION('',(0.,1.,0.));
#17644=DIRECTION('center_axis',(0.,0.,1.));
#17645=DIRECTION('ref_axis',(1.,0.,0.));
#17646=DIRECTION('',(-1.,0.,0.));
#17647=DIRECTION('',(1.,0.,0.));
#17648=DIRECTION('',(0.,1.,0.));
#17649=DIRECTION('center_axis',(-0.939692620785908,0.,0.342020143325669));
#17650=DIRECTION('ref_axis',(0.342020143325669,0.,0.939692620785908));
#17651=DIRECTION('',(-0.342020143325669,0.,-0.939692620785908));
#17652=DIRECTION('',(0.342020143325669,0.,0.939692620785908));
#17653=DIRECTION('',(0.,1.,0.));
#17654=DIRECTION('center_axis',(0.,0.,1.));
#17655=DIRECTION('ref_axis',(1.,0.,0.));
#17656=DIRECTION('',(-1.,0.,0.));
#17657=DIRECTION('',(1.,0.,0.));
#17658=DIRECTION('',(0.,1.,0.));
#17659=DIRECTION('center_axis',(0.939692620785908,0.,0.342020143325669));
#17660=DIRECTION('ref_axis',(0.342020143325669,0.,-0.939692620785908));
#17661=DIRECTION('',(-0.342020143325669,0.,0.939692620785908));
#17662=DIRECTION('',(0.342020143325669,0.,-0.939692620785908));
#17663=DIRECTION('',(0.,1.,0.));
#17664=DIRECTION('center_axis',(0.,0.,1.));
#17665=DIRECTION('ref_axis',(1.,0.,0.));
#17666=DIRECTION('',(-1.,0.,0.));
#17667=DIRECTION('',(1.,0.,0.));
#17668=DIRECTION('',(0.,1.,0.));
#17669=DIRECTION('center_axis',(-0.93969262078591,0.,0.342020143325665));
#17670=DIRECTION('ref_axis',(0.342020143325665,0.,0.93969262078591));
#17671=DIRECTION('',(-0.342020143325665,0.,-0.93969262078591));
#17672=DIRECTION('',(0.342020143325665,0.,0.93969262078591));
#17673=DIRECTION('',(0.,1.,0.));
#17674=DIRECTION('center_axis',(0.,0.,1.));
#17675=DIRECTION('ref_axis',(1.,0.,0.));
#17676=DIRECTION('',(-1.,0.,0.));
#17677=DIRECTION('',(1.,0.,0.));
#17678=DIRECTION('',(0.,1.,0.));
#17679=DIRECTION('center_axis',(0.93969262078591,0.,0.342020143325665));
#17680=DIRECTION('ref_axis',(0.342020143325665,0.,-0.93969262078591));
#17681=DIRECTION('',(-0.342020143325665,0.,0.93969262078591));
#17682=DIRECTION('',(0.342020143325665,0.,-0.93969262078591));
#17683=DIRECTION('',(0.,1.,0.));
#17684=DIRECTION('center_axis',(0.,0.,1.));
#17685=DIRECTION('ref_axis',(1.,0.,0.));
#17686=DIRECTION('',(-1.,0.,0.));
#17687=DIRECTION('',(1.,0.,0.));
#17688=DIRECTION('',(0.,1.,0.));
#17689=DIRECTION('center_axis',(-0.93969262078591,0.,0.342020143325665));
#17690=DIRECTION('ref_axis',(0.342020143325665,0.,0.93969262078591));
#17691=DIRECTION('',(-0.342020143325665,0.,-0.93969262078591));
#17692=DIRECTION('',(0.342020143325665,0.,0.93969262078591));
#17693=DIRECTION('',(0.,1.,0.));
#17694=DIRECTION('center_axis',(0.,0.,1.));
#17695=DIRECTION('ref_axis',(1.,0.,0.));
#17696=DIRECTION('',(-1.,0.,0.));
#17697=DIRECTION('',(1.,0.,0.));
#17698=DIRECTION('',(0.,1.,0.));
#17699=DIRECTION('center_axis',(0.939692620785908,0.,0.342020143325669));
#17700=DIRECTION('ref_axis',(0.342020143325669,0.,-0.939692620785908));
#17701=DIRECTION('',(-0.342020143325669,0.,0.939692620785908));
#17702=DIRECTION('',(0.342020143325669,0.,-0.939692620785908));
#17703=DIRECTION('',(0.,1.,0.));
#17704=DIRECTION('center_axis',(0.,0.,1.));
#17705=DIRECTION('ref_axis',(1.,0.,0.));
#17706=DIRECTION('',(-1.,0.,0.));
#17707=DIRECTION('',(1.,0.,0.));
#17708=DIRECTION('',(0.,1.,0.));
#17709=DIRECTION('center_axis',(-0.939692620785908,0.,0.342020143325669));
#17710=DIRECTION('ref_axis',(0.342020143325669,0.,0.939692620785908));
#17711=DIRECTION('',(-0.342020143325669,0.,-0.939692620785908));
#17712=DIRECTION('',(0.342020143325669,0.,0.939692620785908));
#17713=DIRECTION('',(0.,1.,0.));
#17714=DIRECTION('center_axis',(0.,0.,1.));
#17715=DIRECTION('ref_axis',(1.,0.,0.));
#17716=DIRECTION('',(-1.,0.,0.));
#17717=DIRECTION('',(1.,0.,0.));
#17718=DIRECTION('',(0.,1.,0.));
#17719=DIRECTION('center_axis',(0.93969262078591,0.,0.342020143325665));
#17720=DIRECTION('ref_axis',(0.342020143325665,0.,-0.93969262078591));
#17721=DIRECTION('',(-0.342020143325665,0.,0.93969262078591));
#17722=DIRECTION('',(0.342020143325665,0.,-0.93969262078591));
#17723=DIRECTION('',(0.,1.,0.));
#17724=DIRECTION('center_axis',(0.,0.,1.));
#17725=DIRECTION('ref_axis',(1.,0.,0.));
#17726=DIRECTION('',(-1.,0.,0.));
#17727=DIRECTION('',(1.,0.,0.));
#17728=DIRECTION('',(0.,1.,0.));
#17729=DIRECTION('center_axis',(-0.939692620785907,0.,0.342020143325672));
#17730=DIRECTION('ref_axis',(0.342020143325672,0.,0.939692620785907));
#17731=DIRECTION('',(-0.342020143325672,0.,-0.939692620785907));
#17732=DIRECTION('',(0.342020143325672,0.,0.939692620785907));
#17733=DIRECTION('',(0.,1.,0.));
#17734=DIRECTION('center_axis',(0.,0.,1.));
#17735=DIRECTION('ref_axis',(1.,0.,0.));
#17736=DIRECTION('',(-1.,0.,0.));
#17737=DIRECTION('',(1.,0.,0.));
#17738=DIRECTION('',(0.,1.,0.));
#17739=DIRECTION('center_axis',(0.939692620785907,0.,0.342020143325672));
#17740=DIRECTION('ref_axis',(0.342020143325672,0.,-0.939692620785907));
#17741=DIRECTION('',(-0.342020143325672,0.,0.939692620785907));
#17742=DIRECTION('',(0.342020143325672,0.,-0.939692620785907));
#17743=DIRECTION('',(0.,1.,0.));
#17744=DIRECTION('center_axis',(0.,0.,1.));
#17745=DIRECTION('ref_axis',(1.,0.,0.));
#17746=DIRECTION('',(-1.,0.,0.));
#17747=DIRECTION('',(1.,0.,0.));
#17748=DIRECTION('',(0.,1.,0.));
#17749=DIRECTION('center_axis',(-0.939692620785908,0.,0.342020143325669));
#17750=DIRECTION('ref_axis',(0.342020143325669,0.,0.939692620785908));
#17751=DIRECTION('',(-0.342020143325669,0.,-0.939692620785908));
#17752=DIRECTION('',(0.342020143325669,0.,0.939692620785908));
#17753=DIRECTION('',(0.,1.,0.));
#17754=DIRECTION('center_axis',(0.,0.,1.));
#17755=DIRECTION('ref_axis',(1.,0.,0.));
#17756=DIRECTION('',(-1.,0.,0.));
#17757=DIRECTION('',(1.,0.,0.));
#17758=DIRECTION('',(0.,1.,0.));
#17759=DIRECTION('center_axis',(0.939692620785908,0.,0.342020143325669));
#17760=DIRECTION('ref_axis',(0.342020143325669,0.,-0.939692620785908));
#17761=DIRECTION('',(-0.342020143325669,0.,0.939692620785908));
#17762=DIRECTION('',(0.342020143325669,0.,-0.939692620785908));
#17763=DIRECTION('',(0.,1.,0.));
#17764=DIRECTION('center_axis',(0.,0.,1.));
#17765=DIRECTION('ref_axis',(1.,0.,0.));
#17766=DIRECTION('',(-1.,0.,0.));
#17767=DIRECTION('',(1.,0.,0.));
#17768=DIRECTION('',(0.,1.,0.));
#17769=DIRECTION('center_axis',(-0.939692620785907,0.,0.342020143325672));
#17770=DIRECTION('ref_axis',(0.342020143325672,0.,0.939692620785907));
#17771=DIRECTION('',(-0.342020143325672,0.,-0.939692620785907));
#17772=DIRECTION('',(0.342020143325672,0.,0.939692620785907));
#17773=DIRECTION('',(0.,1.,0.));
#17774=DIRECTION('center_axis',(0.,0.,1.));
#17775=DIRECTION('ref_axis',(1.,0.,0.));
#17776=DIRECTION('',(-1.,0.,0.));
#17777=DIRECTION('',(1.,0.,0.));
#17778=DIRECTION('',(0.,1.,0.));
#17779=DIRECTION('center_axis',(0.939692620785907,0.,0.342020143325672));
#17780=DIRECTION('ref_axis',(0.342020143325672,0.,-0.939692620785907));
#17781=DIRECTION('',(-0.342020143325672,0.,0.939692620785907));
#17782=DIRECTION('',(0.342020143325672,0.,-0.939692620785907));
#17783=DIRECTION('',(0.,1.,0.));
#17784=DIRECTION('center_axis',(0.,0.,1.));
#17785=DIRECTION('ref_axis',(1.,0.,0.));
#17786=DIRECTION('',(-1.,0.,0.));
#17787=DIRECTION('',(1.,0.,0.));
#17788=DIRECTION('',(0.,1.,0.));
#17789=DIRECTION('center_axis',(-0.939692620785908,0.,0.342020143325669));
#17790=DIRECTION('ref_axis',(0.342020143325669,0.,0.939692620785908));
#17791=DIRECTION('',(-0.342020143325669,0.,-0.939692620785908));
#17792=DIRECTION('',(0.342020143325669,0.,0.939692620785908));
#17793=DIRECTION('',(0.,1.,0.));
#17794=DIRECTION('center_axis',(0.,0.,1.));
#17795=DIRECTION('ref_axis',(1.,0.,0.));
#17796=DIRECTION('',(-1.,0.,0.));
#17797=DIRECTION('',(1.,0.,0.));
#17798=DIRECTION('',(0.,1.,0.));
#17799=DIRECTION('center_axis',(0.939692620785908,0.,0.342020143325669));
#17800=DIRECTION('ref_axis',(0.342020143325669,0.,-0.939692620785908));
#17801=DIRECTION('',(-0.342020143325669,0.,0.939692620785908));
#17802=DIRECTION('',(0.342020143325669,0.,-0.939692620785908));
#17803=DIRECTION('',(0.,1.,0.));
#17804=DIRECTION('center_axis',(0.,0.,1.));
#17805=DIRECTION('ref_axis',(1.,0.,0.));
#17806=DIRECTION('',(-1.,0.,0.));
#17807=DIRECTION('',(1.,0.,0.));
#17808=DIRECTION('',(0.,1.,0.));
#17809=DIRECTION('center_axis',(-0.939692620785907,0.,0.342020143325672));
#17810=DIRECTION('ref_axis',(0.342020143325672,0.,0.939692620785907));
#17811=DIRECTION('',(-0.342020143325672,0.,-0.939692620785907));
#17812=DIRECTION('',(0.342020143325672,0.,0.939692620785907));
#17813=DIRECTION('',(0.,1.,0.));
#17814=DIRECTION('center_axis',(0.,0.,1.));
#17815=DIRECTION('ref_axis',(1.,0.,0.));
#17816=DIRECTION('',(-1.,0.,0.));
#17817=DIRECTION('',(1.,0.,0.));
#17818=DIRECTION('',(0.,1.,0.));
#17819=DIRECTION('center_axis',(0.939692620785907,0.,0.342020143325672));
#17820=DIRECTION('ref_axis',(0.342020143325672,0.,-0.939692620785907));
#17821=DIRECTION('',(-0.342020143325672,0.,0.939692620785907));
#17822=DIRECTION('',(0.342020143325672,0.,-0.939692620785907));
#17823=DIRECTION('',(0.,1.,0.));
#17824=DIRECTION('center_axis',(0.,0.,1.));
#17825=DIRECTION('ref_axis',(1.,0.,0.));
#17826=DIRECTION('',(-1.,0.,0.));
#17827=DIRECTION('',(1.,0.,0.));
#17828=DIRECTION('',(0.,1.,0.));
#17829=DIRECTION('center_axis',(-0.939692620785908,0.,0.342020143325669));
#17830=DIRECTION('ref_axis',(0.342020143325669,0.,0.939692620785908));
#17831=DIRECTION('',(-0.342020143325669,0.,-0.939692620785908));
#17832=DIRECTION('',(0.342020143325669,0.,0.939692620785908));
#17833=DIRECTION('',(0.,1.,0.));
#17834=DIRECTION('center_axis',(0.,0.,1.));
#17835=DIRECTION('ref_axis',(1.,0.,0.));
#17836=DIRECTION('',(-1.,0.,0.));
#17837=DIRECTION('',(1.,0.,0.));
#17838=DIRECTION('',(0.,1.,0.));
#17839=DIRECTION('center_axis',(0.939692620785908,0.,0.342020143325669));
#17840=DIRECTION('ref_axis',(0.342020143325669,0.,-0.939692620785908));
#17841=DIRECTION('',(-0.342020143325669,0.,0.939692620785908));
#17842=DIRECTION('',(0.342020143325669,0.,-0.939692620785908));
#17843=DIRECTION('',(0.,1.,0.));
#17844=DIRECTION('center_axis',(0.,0.,1.));
#17845=DIRECTION('ref_axis',(1.,0.,0.));
#17846=DIRECTION('',(-1.,0.,0.));
#17847=DIRECTION('',(1.,0.,0.));
#17848=DIRECTION('',(0.,1.,0.));
#17849=DIRECTION('center_axis',(-0.939692620785907,0.,0.342020143325672));
#17850=DIRECTION('ref_axis',(0.342020143325672,0.,0.939692620785907));
#17851=DIRECTION('',(-0.342020143325672,0.,-0.939692620785907));
#17852=DIRECTION('',(0.342020143325672,0.,0.939692620785907));
#17853=DIRECTION('',(0.,1.,0.));
#17854=DIRECTION('center_axis',(0.,0.,1.));
#17855=DIRECTION('ref_axis',(1.,0.,0.));
#17856=DIRECTION('',(-1.,0.,0.));
#17857=DIRECTION('',(1.,0.,0.));
#17858=DIRECTION('',(0.,1.,0.));
#17859=DIRECTION('center_axis',(0.939692620785907,0.,0.342020143325672));
#17860=DIRECTION('ref_axis',(0.342020143325672,0.,-0.939692620785907));
#17861=DIRECTION('',(-0.342020143325672,0.,0.939692620785907));
#17862=DIRECTION('',(0.342020143325672,0.,-0.939692620785907));
#17863=DIRECTION('',(0.,1.,0.));
#17864=DIRECTION('center_axis',(0.,0.,1.));
#17865=DIRECTION('ref_axis',(1.,0.,0.));
#17866=DIRECTION('',(-1.,0.,0.));
#17867=DIRECTION('',(1.,0.,0.));
#17868=DIRECTION('',(0.,1.,0.));
#17869=DIRECTION('center_axis',(-0.939692620785908,0.,0.34202014332567));
#17870=DIRECTION('ref_axis',(0.34202014332567,0.,0.939692620785908));
#17871=DIRECTION('',(-0.34202014332567,0.,-0.939692620785908));
#17872=DIRECTION('',(0.34202014332567,0.,0.939692620785908));
#17873=DIRECTION('',(0.,1.,0.));
#17874=DIRECTION('center_axis',(0.,0.,1.));
#17875=DIRECTION('ref_axis',(1.,0.,0.));
#17876=DIRECTION('',(-1.,0.,0.));
#17877=DIRECTION('',(1.,0.,0.));
#17878=DIRECTION('',(0.,1.,0.));
#17879=DIRECTION('center_axis',(0.939692620785908,0.,0.342020143325669));
#17880=DIRECTION('ref_axis',(0.342020143325669,0.,-0.939692620785908));
#17881=DIRECTION('',(-0.342020143325669,0.,0.939692620785908));
#17882=DIRECTION('',(0.342020143325669,0.,-0.939692620785908));
#17883=DIRECTION('',(0.,1.,0.));
#17884=DIRECTION('center_axis',(0.,0.,1.));
#17885=DIRECTION('ref_axis',(1.,0.,0.));
#17886=DIRECTION('',(-1.,0.,0.));
#17887=DIRECTION('',(1.,0.,0.));
#17888=DIRECTION('',(0.,1.,0.));
#17889=DIRECTION('center_axis',(-0.939692620785908,0.,0.34202014332567));
#17890=DIRECTION('ref_axis',(0.34202014332567,0.,0.939692620785908));
#17891=DIRECTION('',(-0.34202014332567,0.,-0.939692620785908));
#17892=DIRECTION('',(0.34202014332567,0.,0.939692620785908));
#17893=DIRECTION('',(0.,1.,0.));
#17894=DIRECTION('center_axis',(0.,0.,1.));
#17895=DIRECTION('ref_axis',(1.,0.,0.));
#17896=DIRECTION('',(-1.,0.,0.));
#17897=DIRECTION('',(1.,0.,0.));
#17898=DIRECTION('',(0.,1.,0.));
#17899=DIRECTION('center_axis',(0.939692620785908,0.,0.34202014332567));
#17900=DIRECTION('ref_axis',(0.34202014332567,0.,-0.939692620785908));
#17901=DIRECTION('',(-0.34202014332567,0.,0.939692620785908));
#17902=DIRECTION('',(0.34202014332567,0.,-0.939692620785908));
#17903=DIRECTION('',(0.,1.,0.));
#17904=DIRECTION('center_axis',(0.,0.,1.));
#17905=DIRECTION('ref_axis',(1.,0.,0.));
#17906=DIRECTION('',(-1.,0.,0.));
#17907=DIRECTION('',(1.,0.,0.));
#17908=DIRECTION('',(0.,1.,0.));
#17909=DIRECTION('center_axis',(-0.939692620785908,0.,0.342020143325669));
#17910=DIRECTION('ref_axis',(0.342020143325669,0.,0.939692620785908));
#17911=DIRECTION('',(-0.342020143325669,0.,-0.939692620785908));
#17912=DIRECTION('',(0.342020143325669,0.,0.939692620785908));
#17913=DIRECTION('',(0.,1.,0.));
#17914=DIRECTION('center_axis',(0.,0.,1.));
#17915=DIRECTION('ref_axis',(1.,0.,0.));
#17916=DIRECTION('',(-1.,0.,0.));
#17917=DIRECTION('',(1.,0.,0.));
#17918=DIRECTION('',(0.,1.,0.));
#17919=DIRECTION('center_axis',(0.939692620785908,0.,0.342020143325669));
#17920=DIRECTION('ref_axis',(0.342020143325669,0.,-0.939692620785908));
#17921=DIRECTION('',(-0.342020143325669,0.,0.939692620785908));
#17922=DIRECTION('',(0.342020143325669,0.,-0.939692620785908));
#17923=DIRECTION('',(0.,1.,0.));
#17924=DIRECTION('center_axis',(0.,0.,1.));
#17925=DIRECTION('ref_axis',(1.,0.,0.));
#17926=DIRECTION('',(-1.,0.,0.));
#17927=DIRECTION('',(1.,0.,0.));
#17928=DIRECTION('',(0.,1.,0.));
#17929=DIRECTION('center_axis',(-0.939692620785908,0.,0.34202014332567));
#17930=DIRECTION('ref_axis',(0.34202014332567,0.,0.939692620785908));
#17931=DIRECTION('',(-0.34202014332567,0.,-0.939692620785908));
#17932=DIRECTION('',(0.34202014332567,0.,0.939692620785908));
#17933=DIRECTION('',(0.,1.,0.));
#17934=DIRECTION('center_axis',(0.,0.,1.));
#17935=DIRECTION('ref_axis',(1.,0.,0.));
#17936=DIRECTION('',(-1.,0.,0.));
#17937=DIRECTION('',(1.,0.,0.));
#17938=DIRECTION('',(0.,1.,0.));
#17939=DIRECTION('center_axis',(0.939692620785908,0.,0.342020143325669));
#17940=DIRECTION('ref_axis',(0.342020143325669,0.,-0.939692620785908));
#17941=DIRECTION('',(-0.342020143325669,0.,0.939692620785908));
#17942=DIRECTION('',(0.342020143325669,0.,-0.939692620785908));
#17943=DIRECTION('',(0.,1.,0.));
#17944=DIRECTION('center_axis',(0.,0.,1.));
#17945=DIRECTION('ref_axis',(1.,0.,0.));
#17946=DIRECTION('',(-1.,0.,0.));
#17947=DIRECTION('',(1.,0.,0.));
#17948=DIRECTION('',(0.,1.,0.));
#17949=DIRECTION('center_axis',(-0.939692620785908,0.,0.34202014332567));
#17950=DIRECTION('ref_axis',(0.34202014332567,0.,0.939692620785908));
#17951=DIRECTION('',(-0.34202014332567,0.,-0.939692620785908));
#17952=DIRECTION('',(0.34202014332567,0.,0.939692620785908));
#17953=DIRECTION('',(0.,1.,0.));
#17954=DIRECTION('center_axis',(0.,0.,1.));
#17955=DIRECTION('ref_axis',(1.,0.,0.));
#17956=DIRECTION('',(-1.,0.,0.));
#17957=DIRECTION('',(1.,0.,0.));
#17958=DIRECTION('',(0.,1.,0.));
#17959=DIRECTION('center_axis',(0.939692620785908,0.,0.342020143325669));
#17960=DIRECTION('ref_axis',(0.342020143325669,0.,-0.939692620785908));
#17961=DIRECTION('',(-0.342020143325669,0.,0.939692620785908));
#17962=DIRECTION('',(0.342020143325669,0.,-0.939692620785908));
#17963=DIRECTION('',(0.,1.,0.));
#17964=DIRECTION('center_axis',(0.,0.,1.));
#17965=DIRECTION('ref_axis',(1.,0.,0.));
#17966=DIRECTION('',(-1.,0.,0.));
#17967=DIRECTION('',(1.,0.,0.));
#17968=DIRECTION('',(0.,1.,0.));
#17969=DIRECTION('center_axis',(-0.939692620785908,0.,0.34202014332567));
#17970=DIRECTION('ref_axis',(0.34202014332567,0.,0.939692620785908));
#17971=DIRECTION('',(-0.34202014332567,0.,-0.939692620785908));
#17972=DIRECTION('',(0.34202014332567,0.,0.939692620785908));
#17973=DIRECTION('',(0.,1.,0.));
#17974=DIRECTION('center_axis',(0.,0.,1.));
#17975=DIRECTION('ref_axis',(1.,0.,0.));
#17976=DIRECTION('',(-1.,0.,0.));
#17977=DIRECTION('',(1.,0.,0.));
#17978=DIRECTION('',(0.,1.,0.));
#17979=DIRECTION('center_axis',(0.939692620785908,0.,0.34202014332567));
#17980=DIRECTION('ref_axis',(0.34202014332567,0.,-0.939692620785908));
#17981=DIRECTION('',(-0.34202014332567,0.,0.939692620785908));
#17982=DIRECTION('',(0.34202014332567,0.,-0.939692620785908));
#17983=DIRECTION('',(0.,1.,0.));
#17984=DIRECTION('center_axis',(0.,0.,1.));
#17985=DIRECTION('ref_axis',(1.,0.,0.));
#17986=DIRECTION('',(-1.,0.,0.));
#17987=DIRECTION('',(1.,0.,0.));
#17988=DIRECTION('',(0.,1.,0.));
#17989=DIRECTION('center_axis',(-0.939692620785908,0.,0.34202014332567));
#17990=DIRECTION('ref_axis',(0.34202014332567,0.,0.939692620785908));
#17991=DIRECTION('',(-0.34202014332567,0.,-0.939692620785908));
#17992=DIRECTION('',(0.34202014332567,0.,0.939692620785908));
#17993=DIRECTION('',(0.,1.,0.));
#17994=DIRECTION('center_axis',(0.,0.,1.));
#17995=DIRECTION('ref_axis',(1.,0.,0.));
#17996=DIRECTION('',(-1.,0.,0.));
#17997=DIRECTION('',(1.,0.,0.));
#17998=DIRECTION('',(0.,1.,0.));
#17999=DIRECTION('center_axis',(0.939692620785908,0.,0.342020143325669));
#18000=DIRECTION('ref_axis',(0.342020143325669,0.,-0.939692620785908));
#18001=DIRECTION('',(-0.342020143325669,0.,0.939692620785908));
#18002=DIRECTION('',(0.342020143325669,0.,-0.939692620785908));
#18003=DIRECTION('',(0.,1.,0.));
#18004=DIRECTION('center_axis',(0.,0.,1.));
#18005=DIRECTION('ref_axis',(1.,0.,0.));
#18006=DIRECTION('',(-1.,0.,0.));
#18007=DIRECTION('',(1.,0.,0.));
#18008=DIRECTION('',(0.,1.,0.));
#18009=DIRECTION('center_axis',(-0.939692620785908,0.,0.342020143325669));
#18010=DIRECTION('ref_axis',(0.342020143325669,0.,0.939692620785908));
#18011=DIRECTION('',(-0.342020143325669,0.,-0.939692620785908));
#18012=DIRECTION('',(0.342020143325669,0.,0.939692620785908));
#18013=DIRECTION('',(0.,1.,0.));
#18014=DIRECTION('center_axis',(0.,0.,1.));
#18015=DIRECTION('ref_axis',(1.,0.,0.));
#18016=DIRECTION('',(-1.,0.,0.));
#18017=DIRECTION('',(1.,0.,0.));
#18018=DIRECTION('',(0.,1.,0.));
#18019=DIRECTION('center_axis',(0.939692620785908,0.,0.342020143325669));
#18020=DIRECTION('ref_axis',(0.342020143325669,0.,-0.939692620785908));
#18021=DIRECTION('',(-0.342020143325669,0.,0.939692620785908));
#18022=DIRECTION('',(0.342020143325669,0.,-0.939692620785908));
#18023=DIRECTION('',(0.,1.,0.));
#18024=DIRECTION('center_axis',(0.,0.,1.));
#18025=DIRECTION('ref_axis',(1.,0.,0.));
#18026=DIRECTION('',(-1.,0.,0.));
#18027=DIRECTION('',(1.,0.,0.));
#18028=DIRECTION('',(0.,1.,0.));
#18029=DIRECTION('center_axis',(-0.939692620785908,0.,0.342020143325669));
#18030=DIRECTION('ref_axis',(0.342020143325669,0.,0.939692620785908));
#18031=DIRECTION('',(-0.342020143325669,0.,-0.939692620785908));
#18032=DIRECTION('',(0.342020143325669,0.,0.939692620785908));
#18033=DIRECTION('',(0.,1.,0.));
#18034=DIRECTION('center_axis',(0.,0.,1.));
#18035=DIRECTION('ref_axis',(1.,0.,0.));
#18036=DIRECTION('',(-1.,0.,0.));
#18037=DIRECTION('',(1.,0.,0.));
#18038=DIRECTION('',(0.,1.,0.));
#18039=DIRECTION('center_axis',(0.939692620785908,0.,0.342020143325669));
#18040=DIRECTION('ref_axis',(0.342020143325669,0.,-0.939692620785908));
#18041=DIRECTION('',(-0.342020143325669,0.,0.939692620785908));
#18042=DIRECTION('',(0.342020143325669,0.,-0.939692620785908));
#18043=DIRECTION('',(0.,1.,0.));
#18044=DIRECTION('center_axis',(0.,0.,1.));
#18045=DIRECTION('ref_axis',(1.,0.,0.));
#18046=DIRECTION('',(-1.,0.,0.));
#18047=DIRECTION('',(1.,0.,0.));
#18048=DIRECTION('',(0.,1.,0.));
#18049=DIRECTION('center_axis',(-0.939692620785908,0.,0.342020143325669));
#18050=DIRECTION('ref_axis',(0.342020143325669,0.,0.939692620785908));
#18051=DIRECTION('',(-0.342020143325669,0.,-0.939692620785908));
#18052=DIRECTION('',(0.342020143325669,0.,0.939692620785908));
#18053=DIRECTION('',(0.,1.,0.));
#18054=DIRECTION('center_axis',(0.,0.,1.));
#18055=DIRECTION('ref_axis',(1.,0.,0.));
#18056=DIRECTION('',(-1.,0.,0.));
#18057=DIRECTION('',(1.,0.,0.));
#18058=DIRECTION('',(0.,1.,0.));
#18059=DIRECTION('center_axis',(0.939692620785908,0.,0.342020143325669));
#18060=DIRECTION('ref_axis',(0.342020143325669,0.,-0.939692620785908));
#18061=DIRECTION('',(-0.342020143325669,0.,0.939692620785908));
#18062=DIRECTION('',(0.342020143325669,0.,-0.939692620785908));
#18063=DIRECTION('',(0.,1.,0.));
#18064=DIRECTION('center_axis',(0.,0.,1.));
#18065=DIRECTION('ref_axis',(1.,0.,0.));
#18066=DIRECTION('',(-1.,0.,0.));
#18067=DIRECTION('',(1.,0.,0.));
#18068=DIRECTION('',(0.,1.,0.));
#18069=DIRECTION('center_axis',(-0.939692620785908,0.,0.342020143325669));
#18070=DIRECTION('ref_axis',(0.342020143325669,0.,0.939692620785908));
#18071=DIRECTION('',(-0.342020143325669,0.,-0.939692620785908));
#18072=DIRECTION('',(0.342020143325669,0.,0.939692620785908));
#18073=DIRECTION('',(0.,1.,0.));
#18074=DIRECTION('center_axis',(0.,0.,1.));
#18075=DIRECTION('ref_axis',(1.,0.,0.));
#18076=DIRECTION('',(-1.,0.,0.));
#18077=DIRECTION('',(1.,0.,0.));
#18078=DIRECTION('center_axis',(0.,1.,0.));
#18079=DIRECTION('ref_axis',(0.,0.,1.));
#18080=DIRECTION('center_axis',(0.,1.,0.));
#18081=DIRECTION('ref_axis',(1.,0.,0.));
#21454=CARTESIAN_POINT('',(0.,0.,0.));
#21455=CARTESIAN_POINT('Origin',(17.,-0.6,6.9));
#21456=CARTESIAN_POINT('',(16.835,-0.6,7.));
#21457=CARTESIAN_POINT('Origin',(17.,-0.6,7.));
#21458=CARTESIAN_POINT('',(16.835,-0.6,7.9));
#21459=CARTESIAN_POINT('',(16.835,-0.6,6.9));
#21460=CARTESIAN_POINT('Origin',(17.,-0.6,7.9));
#21461=CARTESIAN_POINT('Origin',(17.,-0.6,7.9));
#21462=CARTESIAN_POINT('Origin',(5.,0.6,6.9));
#21463=CARTESIAN_POINT('',(4.835,0.6,7.));
#21464=CARTESIAN_POINT('Origin',(5.,0.6,7.));
#21465=CARTESIAN_POINT('',(4.835,0.6,7.9));
#21466=CARTESIAN_POINT('',(4.835,0.6,6.9));
#21467=CARTESIAN_POINT('Origin',(5.,0.6,7.9));
#21468=CARTESIAN_POINT('Origin',(5.,0.6,7.9));
#21469=CARTESIAN_POINT('Origin',(5.,-0.6,6.9));
#21470=CARTESIAN_POINT('',(4.835,-0.6,7.));
#21471=CARTESIAN_POINT('Origin',(5.,-0.6,7.));
#21472=CARTESIAN_POINT('',(4.835,-0.6,7.9));
#21473=CARTESIAN_POINT('',(4.835,-0.6,6.9));
#21474=CARTESIAN_POINT('Origin',(5.,-0.6,7.9));
#21475=CARTESIAN_POINT('Origin',(5.,-0.6,7.9));
#21476=CARTESIAN_POINT('Origin',(17.,0.6,6.9));
#21477=CARTESIAN_POINT('',(16.835,0.6,7.));
#21478=CARTESIAN_POINT('Origin',(17.,0.6,7.));
#21479=CARTESIAN_POINT('',(16.835,0.6,7.9));
#21480=CARTESIAN_POINT('',(16.835,0.6,6.9));
#21481=CARTESIAN_POINT('Origin',(17.,0.6,7.9));
#21482=CARTESIAN_POINT('Origin',(17.,0.6,7.9));
#21483=CARTESIAN_POINT('Origin',(1.,-1.,7.));
#21484=CARTESIAN_POINT('',(1.,-1.,8.));
#21485=CARTESIAN_POINT('',(1.,-1.,7.));
#21486=CARTESIAN_POINT('',(1.,-1.,8.));
#21487=CARTESIAN_POINT('',(1.,1.,8.));
#21488=CARTESIAN_POINT('',(1.,-1.,8.));
#21489=CARTESIAN_POINT('',(1.,1.,7.));
#21490=CARTESIAN_POINT('',(1.,1.,8.));
#21491=CARTESIAN_POINT('',(1.,-1.,7.));
#21492=CARTESIAN_POINT('Origin',(21.,-1.,7.));
#21493=CARTESIAN_POINT('',(21.,-1.,7.));
#21494=CARTESIAN_POINT('',(1.,-1.,7.));
#21495=CARTESIAN_POINT('',(21.,1.,7.));
#21496=CARTESIAN_POINT('',(1.,1.,7.));
#21497=CARTESIAN_POINT('',(21.,-1.,7.));
#21498=CARTESIAN_POINT('Origin',(21.,-1.,8.));
#21499=CARTESIAN_POINT('',(21.,-1.,8.));
#21500=CARTESIAN_POINT('',(21.,-1.,7.));
#21501=CARTESIAN_POINT('',(21.,1.,8.));
#21502=CARTESIAN_POINT('',(21.,1.,7.));
#21503=CARTESIAN_POINT('',(21.,-1.,8.));
#21504=CARTESIAN_POINT('Origin',(20.9860094173744,-1.,8.));
#21505=CARTESIAN_POINT('',(20.9860094173744,-1.,8.));
#21506=CARTESIAN_POINT('',(21.,-1.,8.));
#21507=CARTESIAN_POINT('',(20.9860094173744,1.,8.));
#21508=CARTESIAN_POINT('',(21.,1.,8.));
#21509=CARTESIAN_POINT('',(20.9860094173744,-1.,8.));
#21510=CARTESIAN_POINT('Origin',(20.8222228119546,-1.,8.45));
#21511=CARTESIAN_POINT('',(20.8222228119546,-1.,8.45));
#21512=CARTESIAN_POINT('',(20.9860094173744,-1.,8.));
#21513=CARTESIAN_POINT('',(20.8222228119546,1.,8.45));
#21514=CARTESIAN_POINT('',(20.9860094173744,1.,8.));
#21515=CARTESIAN_POINT('',(20.8222228119546,-1.,8.45));
#21516=CARTESIAN_POINT('Origin',(20.6556516403021,-1.,8.45));
#21517=CARTESIAN_POINT('',(20.6556516403021,-1.,8.45));
#21518=CARTESIAN_POINT('',(20.8222228119546,-1.,8.45));
#21519=CARTESIAN_POINT('',(20.6556516403021,1.,8.45));
#21520=CARTESIAN_POINT('',(20.8222228119546,1.,8.45));
#21521=CARTESIAN_POINT('',(20.6556516403021,-1.,8.45));
#21522=CARTESIAN_POINT('Origin',(20.4918650348823,-1.,8.));
#21523=CARTESIAN_POINT('',(20.4918650348823,-1.,8.));
#21524=CARTESIAN_POINT('',(20.6556516403021,-1.,8.45));
#21525=CARTESIAN_POINT('',(20.4918650348823,1.,8.));
#21526=CARTESIAN_POINT('',(20.6556516403021,1.,8.45));
#21527=CARTESIAN_POINT('',(20.4918650348823,-1.,8.));
#21528=CARTESIAN_POINT('Origin',(20.3576908866564,-1.,8.));
#21529=CARTESIAN_POINT('',(20.3576908866564,-1.,8.));
#21530=CARTESIAN_POINT('',(20.4918650348823,-1.,8.));
#21531=CARTESIAN_POINT('',(20.3576908866564,1.,8.));
#21532=CARTESIAN_POINT('',(20.4918650348823,1.,8.));
#21533=CARTESIAN_POINT('',(20.3576908866564,-1.,8.));
#21534=CARTESIAN_POINT('Origin',(20.1939042812366,-1.,8.45));
#21535=CARTESIAN_POINT('',(20.1939042812366,-1.,8.45));
#21536=CARTESIAN_POINT('',(20.3576908866564,-1.,8.));
#21537=CARTESIAN_POINT('',(20.1939042812366,1.,8.45));
#21538=CARTESIAN_POINT('',(20.3576908866564,1.,8.));
#21539=CARTESIAN_POINT('',(20.1939042812366,-1.,8.45));
#21540=CARTESIAN_POINT('Origin',(20.0273331095842,-1.,8.45));
#21541=CARTESIAN_POINT('',(20.0273331095842,-1.,8.45));
#21542=CARTESIAN_POINT('',(20.1939042812366,-1.,8.45));
#21543=CARTESIAN_POINT('',(20.0273331095842,1.,8.45));
#21544=CARTESIAN_POINT('',(20.1939042812366,1.,8.45));
#21545=CARTESIAN_POINT('',(20.0273331095842,-1.,8.45));
#21546=CARTESIAN_POINT('Origin',(19.8635465041644,-1.,8.));
#21547=CARTESIAN_POINT('',(19.8635465041644,-1.,8.));
#21548=CARTESIAN_POINT('',(20.0273331095842,-1.,8.45));
#21549=CARTESIAN_POINT('',(19.8635465041644,1.,8.));
#21550=CARTESIAN_POINT('',(20.0273331095842,1.,8.45));
#21551=CARTESIAN_POINT('',(19.8635465041644,-1.,8.));
#21552=CARTESIAN_POINT('Origin',(19.7293723559385,-1.,8.));
#21553=CARTESIAN_POINT('',(19.7293723559385,-1.,8.));
#21554=CARTESIAN_POINT('',(19.8635465041644,-1.,8.));
#21555=CARTESIAN_POINT('',(19.7293723559385,1.,8.));
#21556=CARTESIAN_POINT('',(19.8635465041644,1.,8.));
#21557=CARTESIAN_POINT('',(19.7293723559385,-1.,8.));
#21558=CARTESIAN_POINT('Origin',(19.5655857505187,-1.,8.45));
#21559=CARTESIAN_POINT('',(19.5655857505187,-1.,8.45));
#21560=CARTESIAN_POINT('',(19.7293723559385,-1.,8.));
#21561=CARTESIAN_POINT('',(19.5655857505187,1.,8.45));
#21562=CARTESIAN_POINT('',(19.7293723559385,1.,8.));
#21563=CARTESIAN_POINT('',(19.5655857505187,-1.,8.45));
#21564=CARTESIAN_POINT('Origin',(19.3990145788662,-1.,8.45));
#21565=CARTESIAN_POINT('',(19.3990145788662,-1.,8.45));
#21566=CARTESIAN_POINT('',(19.5655857505187,-1.,8.45));
#21567=CARTESIAN_POINT('',(19.3990145788662,1.,8.45));
#21568=CARTESIAN_POINT('',(19.5655857505187,1.,8.45));
#21569=CARTESIAN_POINT('',(19.3990145788662,-1.,8.45));
#21570=CARTESIAN_POINT('Origin',(19.2352279734464,-1.,8.));
#21571=CARTESIAN_POINT('',(19.2352279734464,-1.,8.));
#21572=CARTESIAN_POINT('',(19.3990145788662,-1.,8.45));
#21573=CARTESIAN_POINT('',(19.2352279734464,1.,8.));
#21574=CARTESIAN_POINT('',(19.3990145788662,1.,8.45));
#21575=CARTESIAN_POINT('',(19.2352279734464,-1.,8.));
#21576=CARTESIAN_POINT('Origin',(19.1010538252205,-1.,8.));
#21577=CARTESIAN_POINT('',(19.1010538252205,-1.,8.));
#21578=CARTESIAN_POINT('',(19.2352279734464,-1.,8.));
#21579=CARTESIAN_POINT('',(19.1010538252205,1.,8.));
#21580=CARTESIAN_POINT('',(19.2352279734464,1.,8.));
#21581=CARTESIAN_POINT('',(19.1010538252205,-1.,8.));
#21582=CARTESIAN_POINT('Origin',(18.9372672198007,-1.,8.45));
#21583=CARTESIAN_POINT('',(18.9372672198007,-1.,8.45));
#21584=CARTESIAN_POINT('',(19.1010538252205,-1.,8.));
#21585=CARTESIAN_POINT('',(18.9372672198007,1.,8.45));
#21586=CARTESIAN_POINT('',(19.1010538252205,1.,8.));
#21587=CARTESIAN_POINT('',(18.9372672198007,-1.,8.45));
#21588=CARTESIAN_POINT('Origin',(18.7706960481482,-1.,8.45));
#21589=CARTESIAN_POINT('',(18.7706960481482,-1.,8.45));
#21590=CARTESIAN_POINT('',(18.9372672198007,-1.,8.45));
#21591=CARTESIAN_POINT('',(18.7706960481482,1.,8.45));
#21592=CARTESIAN_POINT('',(18.9372672198007,1.,8.45));
#21593=CARTESIAN_POINT('',(18.7706960481482,-1.,8.45));
#21594=CARTESIAN_POINT('Origin',(18.6069094427284,-1.,8.));
#21595=CARTESIAN_POINT('',(18.6069094427284,-1.,8.));
#21596=CARTESIAN_POINT('',(18.7706960481482,-1.,8.45));
#21597=CARTESIAN_POINT('',(18.6069094427284,1.,8.));
#21598=CARTESIAN_POINT('',(18.7706960481482,1.,8.45));
#21599=CARTESIAN_POINT('',(18.6069094427284,-1.,8.));
#21600=CARTESIAN_POINT('Origin',(18.4727352945026,-1.,8.));
#21601=CARTESIAN_POINT('',(18.4727352945026,-1.,8.));
#21602=CARTESIAN_POINT('',(18.6069094427284,-1.,8.));
#21603=CARTESIAN_POINT('',(18.4727352945026,1.,8.));
#21604=CARTESIAN_POINT('',(18.6069094427284,1.,8.));
#21605=CARTESIAN_POINT('',(18.4727352945026,-1.,8.));
#21606=CARTESIAN_POINT('Origin',(18.3089486890828,-1.,8.45));
#21607=CARTESIAN_POINT('',(18.3089486890828,-1.,8.45));
#21608=CARTESIAN_POINT('',(18.4727352945026,-1.,8.));
#21609=CARTESIAN_POINT('',(18.3089486890828,1.,8.45));
#21610=CARTESIAN_POINT('',(18.4727352945026,1.,8.));
#21611=CARTESIAN_POINT('',(18.3089486890828,-1.,8.45));
#21612=CARTESIAN_POINT('Origin',(18.1423775174303,-1.,8.45));
#21613=CARTESIAN_POINT('',(18.1423775174303,-1.,8.45));
#21614=CARTESIAN_POINT('',(18.3089486890828,-1.,8.45));
#21615=CARTESIAN_POINT('',(18.1423775174303,1.,8.45));
#21616=CARTESIAN_POINT('',(18.3089486890828,1.,8.45));
#21617=CARTESIAN_POINT('',(18.1423775174303,-1.,8.45));
#21618=CARTESIAN_POINT('Origin',(17.9785909120105,-1.,8.));
#21619=CARTESIAN_POINT('',(17.9785909120105,-1.,8.));
#21620=CARTESIAN_POINT('',(18.1423775174303,-1.,8.45));
#21621=CARTESIAN_POINT('',(17.9785909120105,1.,8.));
#21622=CARTESIAN_POINT('',(18.1423775174303,1.,8.45));
#21623=CARTESIAN_POINT('',(17.9785909120105,-1.,8.));
#21624=CARTESIAN_POINT('Origin',(17.8444167637846,-1.,8.));
#21625=CARTESIAN_POINT('',(17.8444167637846,-1.,8.));
#21626=CARTESIAN_POINT('',(17.9785909120105,-1.,8.));
#21627=CARTESIAN_POINT('',(17.8444167637846,1.,8.));
#21628=CARTESIAN_POINT('',(17.9785909120105,1.,8.));
#21629=CARTESIAN_POINT('',(17.8444167637846,-1.,8.));
#21630=CARTESIAN_POINT('Origin',(17.6806301583648,-1.,8.45));
#21631=CARTESIAN_POINT('',(17.6806301583648,-1.,8.45));
#21632=CARTESIAN_POINT('',(17.8444167637846,-1.,8.));
#21633=CARTESIAN_POINT('',(17.6806301583648,1.,8.45));
#21634=CARTESIAN_POINT('',(17.8444167637846,1.,8.));
#21635=CARTESIAN_POINT('',(17.6806301583648,-1.,8.45));
#21636=CARTESIAN_POINT('Origin',(17.5140589867123,-1.,8.45));
#21637=CARTESIAN_POINT('',(17.5140589867123,-1.,8.45));
#21638=CARTESIAN_POINT('',(17.6806301583648,-1.,8.45));
#21639=CARTESIAN_POINT('',(17.5140589867123,1.,8.45));
#21640=CARTESIAN_POINT('',(17.6806301583648,1.,8.45));
#21641=CARTESIAN_POINT('',(17.5140589867123,-1.,8.45));
#21642=CARTESIAN_POINT('Origin',(17.3502723812925,-1.,8.));
#21643=CARTESIAN_POINT('',(17.3502723812925,-1.,8.));
#21644=CARTESIAN_POINT('',(17.5140589867123,-1.,8.45));
#21645=CARTESIAN_POINT('',(17.3502723812925,1.,8.));
#21646=CARTESIAN_POINT('',(17.5140589867123,1.,8.45));
#21647=CARTESIAN_POINT('',(17.3502723812925,-1.,8.));
#21648=CARTESIAN_POINT('Origin',(17.2160982330666,-1.,8.));
#21649=CARTESIAN_POINT('',(17.2160982330666,-1.,8.));
#21650=CARTESIAN_POINT('',(17.3502723812925,-1.,8.));
#21651=CARTESIAN_POINT('',(17.2160982330666,1.,8.));
#21652=CARTESIAN_POINT('',(17.3502723812925,1.,8.));
#21653=CARTESIAN_POINT('',(17.2160982330666,-1.,8.));
#21654=CARTESIAN_POINT('Origin',(17.0523116276469,-1.,8.45));
#21655=CARTESIAN_POINT('',(17.0523116276469,-1.,8.45));
#21656=CARTESIAN_POINT('',(17.2160982330666,-1.,8.));
#21657=CARTESIAN_POINT('',(17.0523116276469,1.,8.45));
#21658=CARTESIAN_POINT('',(17.2160982330666,1.,8.));
#21659=CARTESIAN_POINT('',(17.0523116276469,-1.,8.45));
#21660=CARTESIAN_POINT('Origin',(16.8857404559944,-1.,8.45));
#21661=CARTESIAN_POINT('',(16.8857404559944,-1.,8.45));
#21662=CARTESIAN_POINT('',(17.0523116276469,-1.,8.45));
#21663=CARTESIAN_POINT('',(16.8857404559944,1.,8.45));
#21664=CARTESIAN_POINT('',(17.0523116276469,1.,8.45));
#21665=CARTESIAN_POINT('',(16.8857404559944,-1.,8.45));
#21666=CARTESIAN_POINT('Origin',(16.7219538505746,-1.,8.));
#21667=CARTESIAN_POINT('',(16.7219538505746,-1.,8.));
#21668=CARTESIAN_POINT('',(16.8857404559944,-1.,8.45));
#21669=CARTESIAN_POINT('',(16.7219538505746,1.,8.));
#21670=CARTESIAN_POINT('',(16.8857404559944,1.,8.45));
#21671=CARTESIAN_POINT('',(16.7219538505746,-1.,8.));
#21672=CARTESIAN_POINT('Origin',(16.5877797023487,-1.,8.));
#21673=CARTESIAN_POINT('',(16.5877797023487,-1.,8.));
#21674=CARTESIAN_POINT('',(16.7219538505746,-1.,8.));
#21675=CARTESIAN_POINT('',(16.5877797023487,1.,8.));
#21676=CARTESIAN_POINT('',(16.7219538505746,1.,8.));
#21677=CARTESIAN_POINT('',(16.5877797023487,-1.,8.));
#21678=CARTESIAN_POINT('Origin',(16.4239930969289,-1.,8.45));
#21679=CARTESIAN_POINT('',(16.4239930969289,-1.,8.45));
#21680=CARTESIAN_POINT('',(16.5877797023487,-1.,8.));
#21681=CARTESIAN_POINT('',(16.4239930969289,1.,8.45));
#21682=CARTESIAN_POINT('',(16.5877797023487,1.,8.));
#21683=CARTESIAN_POINT('',(16.4239930969289,-1.,8.45));
#21684=CARTESIAN_POINT('Origin',(16.2574219252764,-1.,8.45));
#21685=CARTESIAN_POINT('',(16.2574219252764,-1.,8.45));
#21686=CARTESIAN_POINT('',(16.4239930969289,-1.,8.45));
#21687=CARTESIAN_POINT('',(16.2574219252764,1.,8.45));
#21688=CARTESIAN_POINT('',(16.4239930969289,1.,8.45));
#21689=CARTESIAN_POINT('',(16.2574219252764,-1.,8.45));
#21690=CARTESIAN_POINT('Origin',(16.0936353198566,-1.,8.));
#21691=CARTESIAN_POINT('',(16.0936353198566,-1.,8.));
#21692=CARTESIAN_POINT('',(16.2574219252764,-1.,8.45));
#21693=CARTESIAN_POINT('',(16.0936353198566,1.,8.));
#21694=CARTESIAN_POINT('',(16.2574219252764,1.,8.45));
#21695=CARTESIAN_POINT('',(16.0936353198566,-1.,8.));
#21696=CARTESIAN_POINT('Origin',(15.9594611716307,-1.,8.));
#21697=CARTESIAN_POINT('',(15.9594611716307,-1.,8.));
#21698=CARTESIAN_POINT('',(16.0936353198566,-1.,8.));
#21699=CARTESIAN_POINT('',(15.9594611716307,1.,8.));
#21700=CARTESIAN_POINT('',(16.0936353198566,1.,8.));
#21701=CARTESIAN_POINT('',(15.9594611716307,-1.,8.));
#21702=CARTESIAN_POINT('Origin',(15.7956745662109,-1.,8.45));
#21703=CARTESIAN_POINT('',(15.7956745662109,-1.,8.45));
#21704=CARTESIAN_POINT('',(15.9594611716307,-1.,8.));
#21705=CARTESIAN_POINT('',(15.7956745662109,1.,8.45));
#21706=CARTESIAN_POINT('',(15.9594611716307,1.,8.));
#21707=CARTESIAN_POINT('',(15.7956745662109,-1.,8.45));
#21708=CARTESIAN_POINT('Origin',(15.6291033945584,-1.,8.45));
#21709=CARTESIAN_POINT('',(15.6291033945584,-1.,8.45));
#21710=CARTESIAN_POINT('',(15.7956745662109,-1.,8.45));
#21711=CARTESIAN_POINT('',(15.6291033945584,1.,8.45));
#21712=CARTESIAN_POINT('',(15.7956745662109,1.,8.45));
#21713=CARTESIAN_POINT('',(15.6291033945584,-1.,8.45));
#21714=CARTESIAN_POINT('Origin',(15.4653167891387,-1.,8.));
#21715=CARTESIAN_POINT('',(15.4653167891387,-1.,8.));
#21716=CARTESIAN_POINT('',(15.6291033945584,-1.,8.45));
#21717=CARTESIAN_POINT('',(15.4653167891387,1.,8.));
#21718=CARTESIAN_POINT('',(15.6291033945584,1.,8.45));
#21719=CARTESIAN_POINT('',(15.4653167891387,-1.,8.));
#21720=CARTESIAN_POINT('Origin',(15.3311426409128,-1.,8.));
#21721=CARTESIAN_POINT('',(15.3311426409128,-1.,8.));
#21722=CARTESIAN_POINT('',(15.4653167891387,-1.,8.));
#21723=CARTESIAN_POINT('',(15.3311426409128,1.,8.));
#21724=CARTESIAN_POINT('',(15.4653167891387,1.,8.));
#21725=CARTESIAN_POINT('',(15.3311426409128,-1.,8.));
#21726=CARTESIAN_POINT('Origin',(15.167356035493,-1.,8.45));
#21727=CARTESIAN_POINT('',(15.167356035493,-1.,8.45));
#21728=CARTESIAN_POINT('',(15.3311426409128,-1.,8.));
#21729=CARTESIAN_POINT('',(15.167356035493,1.,8.45));
#21730=CARTESIAN_POINT('',(15.3311426409128,1.,8.));
#21731=CARTESIAN_POINT('',(15.167356035493,-1.,8.45));
#21732=CARTESIAN_POINT('Origin',(15.0007848638405,-1.,8.45));
#21733=CARTESIAN_POINT('',(15.0007848638405,-1.,8.45));
#21734=CARTESIAN_POINT('',(15.167356035493,-1.,8.45));
#21735=CARTESIAN_POINT('',(15.0007848638405,1.,8.45));
#21736=CARTESIAN_POINT('',(15.167356035493,1.,8.45));
#21737=CARTESIAN_POINT('',(15.0007848638405,-1.,8.45));
#21738=CARTESIAN_POINT('Origin',(14.8369982584207,-1.,8.));
#21739=CARTESIAN_POINT('',(14.8369982584207,-1.,8.));
#21740=CARTESIAN_POINT('',(15.0007848638405,-1.,8.45));
#21741=CARTESIAN_POINT('',(14.8369982584207,1.,8.));
#21742=CARTESIAN_POINT('',(15.0007848638405,1.,8.45));
#21743=CARTESIAN_POINT('',(14.8369982584207,-1.,8.));
#21744=CARTESIAN_POINT('Origin',(14.7028241101948,-1.,8.));
#21745=CARTESIAN_POINT('',(14.7028241101948,-1.,8.));
#21746=CARTESIAN_POINT('',(14.8369982584207,-1.,8.));
#21747=CARTESIAN_POINT('',(14.7028241101948,1.,8.));
#21748=CARTESIAN_POINT('',(14.8369982584207,1.,8.));
#21749=CARTESIAN_POINT('',(14.7028241101948,-1.,8.));
#21750=CARTESIAN_POINT('Origin',(14.539037504775,-1.,8.45));
#21751=CARTESIAN_POINT('',(14.539037504775,-1.,8.45));
#21752=CARTESIAN_POINT('',(14.7028241101948,-1.,8.));
#21753=CARTESIAN_POINT('',(14.539037504775,1.,8.45));
#21754=CARTESIAN_POINT('',(14.7028241101948,1.,8.));
#21755=CARTESIAN_POINT('',(14.539037504775,-1.,8.45));
#21756=CARTESIAN_POINT('Origin',(14.3724663331225,-1.,8.45));
#21757=CARTESIAN_POINT('',(14.3724663331225,-1.,8.45));
#21758=CARTESIAN_POINT('',(14.539037504775,-1.,8.45));
#21759=CARTESIAN_POINT('',(14.3724663331225,1.,8.45));
#21760=CARTESIAN_POINT('',(14.539037504775,1.,8.45));
#21761=CARTESIAN_POINT('',(14.3724663331225,-1.,8.45));
#21762=CARTESIAN_POINT('Origin',(14.2086797277027,-1.,8.));
#21763=CARTESIAN_POINT('',(14.2086797277027,-1.,8.));
#21764=CARTESIAN_POINT('',(14.3724663331225,-1.,8.45));
#21765=CARTESIAN_POINT('',(14.2086797277027,1.,8.));
#21766=CARTESIAN_POINT('',(14.3724663331225,1.,8.45));
#21767=CARTESIAN_POINT('',(14.2086797277027,-1.,8.));
#21768=CARTESIAN_POINT('Origin',(14.0745055794769,-1.,8.));
#21769=CARTESIAN_POINT('',(14.0745055794769,-1.,8.));
#21770=CARTESIAN_POINT('',(14.2086797277027,-1.,8.));
#21771=CARTESIAN_POINT('',(14.0745055794769,1.,8.));
#21772=CARTESIAN_POINT('',(14.2086797277027,1.,8.));
#21773=CARTESIAN_POINT('',(14.0745055794769,-1.,8.));
#21774=CARTESIAN_POINT('Origin',(13.9107189740571,-1.,8.45));
#21775=CARTESIAN_POINT('',(13.9107189740571,-1.,8.45));
#21776=CARTESIAN_POINT('',(14.0745055794769,-1.,8.));
#21777=CARTESIAN_POINT('',(13.9107189740571,1.,8.45));
#21778=CARTESIAN_POINT('',(14.0745055794769,1.,8.));
#21779=CARTESIAN_POINT('',(13.9107189740571,-1.,8.45));
#21780=CARTESIAN_POINT('Origin',(13.7441478024046,-1.,8.45));
#21781=CARTESIAN_POINT('',(13.7441478024046,-1.,8.45));
#21782=CARTESIAN_POINT('',(13.9107189740571,-1.,8.45));
#21783=CARTESIAN_POINT('',(13.7441478024046,1.,8.45));
#21784=CARTESIAN_POINT('',(13.9107189740571,1.,8.45));
#21785=CARTESIAN_POINT('',(13.7441478024046,-1.,8.45));
#21786=CARTESIAN_POINT('Origin',(13.5803611969848,-1.,8.));
#21787=CARTESIAN_POINT('',(13.5803611969848,-1.,8.));
#21788=CARTESIAN_POINT('',(13.7441478024046,-1.,8.45));
#21789=CARTESIAN_POINT('',(13.5803611969848,1.,8.));
#21790=CARTESIAN_POINT('',(13.7441478024046,1.,8.45));
#21791=CARTESIAN_POINT('',(13.5803611969848,-1.,8.));
#21792=CARTESIAN_POINT('Origin',(13.4461870487589,-1.,8.));
#21793=CARTESIAN_POINT('',(13.4461870487589,-1.,8.));
#21794=CARTESIAN_POINT('',(13.5803611969848,-1.,8.));
#21795=CARTESIAN_POINT('',(13.4461870487589,1.,8.));
#21796=CARTESIAN_POINT('',(13.5803611969848,1.,8.));
#21797=CARTESIAN_POINT('',(13.4461870487589,-1.,8.));
#21798=CARTESIAN_POINT('Origin',(13.2824004433391,-1.,8.45));
#21799=CARTESIAN_POINT('',(13.2824004433391,-1.,8.45));
#21800=CARTESIAN_POINT('',(13.4461870487589,-1.,8.));
#21801=CARTESIAN_POINT('',(13.2824004433391,1.,8.45));
#21802=CARTESIAN_POINT('',(13.4461870487589,1.,8.));
#21803=CARTESIAN_POINT('',(13.2824004433391,-1.,8.45));
#21804=CARTESIAN_POINT('Origin',(13.1158292716866,-1.,8.45));
#21805=CARTESIAN_POINT('',(13.1158292716866,-1.,8.45));
#21806=CARTESIAN_POINT('',(13.2824004433391,-1.,8.45));
#21807=CARTESIAN_POINT('',(13.1158292716866,1.,8.45));
#21808=CARTESIAN_POINT('',(13.2824004433391,1.,8.45));
#21809=CARTESIAN_POINT('',(13.1158292716866,-1.,8.45));
#21810=CARTESIAN_POINT('Origin',(12.9520426662668,-1.,8.));
#21811=CARTESIAN_POINT('',(12.9520426662668,-1.,8.));
#21812=CARTESIAN_POINT('',(13.1158292716866,-1.,8.45));
#21813=CARTESIAN_POINT('',(12.9520426662668,1.,8.));
#21814=CARTESIAN_POINT('',(13.1158292716866,1.,8.45));
#21815=CARTESIAN_POINT('',(12.9520426662668,-1.,8.));
#21816=CARTESIAN_POINT('Origin',(12.8178685180409,-1.,8.));
#21817=CARTESIAN_POINT('',(12.8178685180409,-1.,8.));
#21818=CARTESIAN_POINT('',(12.9520426662668,-1.,8.));
#21819=CARTESIAN_POINT('',(12.8178685180409,1.,8.));
#21820=CARTESIAN_POINT('',(12.9520426662668,1.,8.));
#21821=CARTESIAN_POINT('',(12.8178685180409,-1.,8.));
#21822=CARTESIAN_POINT('Origin',(12.6540819126211,-1.,8.45));
#21823=CARTESIAN_POINT('',(12.6540819126211,-1.,8.45));
#21824=CARTESIAN_POINT('',(12.8178685180409,-1.,8.));
#21825=CARTESIAN_POINT('',(12.6540819126211,1.,8.45));
#21826=CARTESIAN_POINT('',(12.8178685180409,1.,8.));
#21827=CARTESIAN_POINT('',(12.6540819126211,-1.,8.45));
#21828=CARTESIAN_POINT('Origin',(12.4875107409686,-1.,8.45));
#21829=CARTESIAN_POINT('',(12.4875107409686,-1.,8.45));
#21830=CARTESIAN_POINT('',(12.6540819126211,-1.,8.45));
#21831=CARTESIAN_POINT('',(12.4875107409686,1.,8.45));
#21832=CARTESIAN_POINT('',(12.6540819126211,1.,8.45));
#21833=CARTESIAN_POINT('',(12.4875107409686,-1.,8.45));
#21834=CARTESIAN_POINT('Origin',(12.3237241355489,-1.,8.));
#21835=CARTESIAN_POINT('',(12.3237241355489,-1.,8.));
#21836=CARTESIAN_POINT('',(12.4875107409686,-1.,8.45));
#21837=CARTESIAN_POINT('',(12.3237241355489,1.,8.));
#21838=CARTESIAN_POINT('',(12.4875107409686,1.,8.45));
#21839=CARTESIAN_POINT('',(12.3237241355489,-1.,8.));
#21840=CARTESIAN_POINT('Origin',(12.189549987323,-1.,8.));
#21841=CARTESIAN_POINT('',(12.189549987323,-1.,8.));
#21842=CARTESIAN_POINT('',(12.3237241355489,-1.,8.));
#21843=CARTESIAN_POINT('',(12.189549987323,1.,8.));
#21844=CARTESIAN_POINT('',(12.3237241355489,1.,8.));
#21845=CARTESIAN_POINT('',(12.189549987323,-1.,8.));
#21846=CARTESIAN_POINT('Origin',(12.0257633819032,-1.,8.45));
#21847=CARTESIAN_POINT('',(12.0257633819032,-1.,8.45));
#21848=CARTESIAN_POINT('',(12.189549987323,-1.,8.));
#21849=CARTESIAN_POINT('',(12.0257633819032,1.,8.45));
#21850=CARTESIAN_POINT('',(12.189549987323,1.,8.));
#21851=CARTESIAN_POINT('',(12.0257633819032,-1.,8.45));
#21852=CARTESIAN_POINT('Origin',(11.8591922102507,-1.,8.45));
#21853=CARTESIAN_POINT('',(11.8591922102507,-1.,8.45));
#21854=CARTESIAN_POINT('',(12.0257633819032,-1.,8.45));
#21855=CARTESIAN_POINT('',(11.8591922102507,1.,8.45));
#21856=CARTESIAN_POINT('',(12.0257633819032,1.,8.45));
#21857=CARTESIAN_POINT('',(11.8591922102507,-1.,8.45));
#21858=CARTESIAN_POINT('Origin',(11.6954056048309,-1.,8.));
#21859=CARTESIAN_POINT('',(11.6954056048309,-1.,8.));
#21860=CARTESIAN_POINT('',(11.8591922102507,-1.,8.45));
#21861=CARTESIAN_POINT('',(11.6954056048309,1.,8.));
#21862=CARTESIAN_POINT('',(11.8591922102507,1.,8.45));
#21863=CARTESIAN_POINT('',(11.6954056048309,-1.,8.));
#21864=CARTESIAN_POINT('Origin',(11.561231456605,-1.,8.));
#21865=CARTESIAN_POINT('',(11.561231456605,-1.,8.));
#21866=CARTESIAN_POINT('',(11.6954056048309,-1.,8.));
#21867=CARTESIAN_POINT('',(11.561231456605,1.,8.));
#21868=CARTESIAN_POINT('',(11.6954056048309,1.,8.));
#21869=CARTESIAN_POINT('',(11.561231456605,-1.,8.));
#21870=CARTESIAN_POINT('Origin',(11.3974448511852,-1.,8.45));
#21871=CARTESIAN_POINT('',(11.3974448511852,-1.,8.45));
#21872=CARTESIAN_POINT('',(11.561231456605,-1.,8.));
#21873=CARTESIAN_POINT('',(11.3974448511852,1.,8.45));
#21874=CARTESIAN_POINT('',(11.561231456605,1.,8.));
#21875=CARTESIAN_POINT('',(11.3974448511852,-1.,8.45));
#21876=CARTESIAN_POINT('Origin',(11.2308736795327,-1.,8.45));
#21877=CARTESIAN_POINT('',(11.2308736795327,-1.,8.45));
#21878=CARTESIAN_POINT('',(11.3974448511852,-1.,8.45));
#21879=CARTESIAN_POINT('',(11.2308736795327,1.,8.45));
#21880=CARTESIAN_POINT('',(11.3974448511852,1.,8.45));
#21881=CARTESIAN_POINT('',(11.2308736795327,-1.,8.45));
#21882=CARTESIAN_POINT('Origin',(11.0670870741129,-1.,8.));
#21883=CARTESIAN_POINT('',(11.0670870741129,-1.,8.));
#21884=CARTESIAN_POINT('',(11.2308736795327,-1.,8.45));
#21885=CARTESIAN_POINT('',(11.0670870741129,1.,8.));
#21886=CARTESIAN_POINT('',(11.2308736795327,1.,8.45));
#21887=CARTESIAN_POINT('',(11.0670870741129,-1.,8.));
#21888=CARTESIAN_POINT('Origin',(10.9329129258871,-1.,8.));
#21889=CARTESIAN_POINT('',(10.9329129258871,-1.,8.));
#21890=CARTESIAN_POINT('',(11.0670870741129,-1.,8.));
#21891=CARTESIAN_POINT('',(10.9329129258871,1.,8.));
#21892=CARTESIAN_POINT('',(11.0670870741129,1.,8.));
#21893=CARTESIAN_POINT('',(10.9329129258871,-1.,8.));
#21894=CARTESIAN_POINT('Origin',(10.7691263204673,-1.,8.45));
#21895=CARTESIAN_POINT('',(10.7691263204673,-1.,8.45));
#21896=CARTESIAN_POINT('',(10.9329129258871,-1.,8.));
#21897=CARTESIAN_POINT('',(10.7691263204673,1.,8.45));
#21898=CARTESIAN_POINT('',(10.9329129258871,1.,8.));
#21899=CARTESIAN_POINT('',(10.7691263204673,-1.,8.45));
#21900=CARTESIAN_POINT('Origin',(10.6025551488148,-1.,8.45));
#21901=CARTESIAN_POINT('',(10.6025551488148,-1.,8.45));
#21902=CARTESIAN_POINT('',(10.7691263204673,-1.,8.45));
#21903=CARTESIAN_POINT('',(10.6025551488148,1.,8.45));
#21904=CARTESIAN_POINT('',(10.7691263204673,1.,8.45));
#21905=CARTESIAN_POINT('',(10.6025551488148,-1.,8.45));
#21906=CARTESIAN_POINT('Origin',(10.438768543395,-1.,8.));
#21907=CARTESIAN_POINT('',(10.438768543395,-1.,8.));
#21908=CARTESIAN_POINT('',(10.6025551488148,-1.,8.45));
#21909=CARTESIAN_POINT('',(10.438768543395,1.,8.));
#21910=CARTESIAN_POINT('',(10.6025551488148,1.,8.45));
#21911=CARTESIAN_POINT('',(10.438768543395,-1.,8.));
#21912=CARTESIAN_POINT('Origin',(10.3045943951691,-1.,8.));
#21913=CARTESIAN_POINT('',(10.3045943951691,-1.,8.));
#21914=CARTESIAN_POINT('',(10.438768543395,-1.,8.));
#21915=CARTESIAN_POINT('',(10.3045943951691,1.,8.));
#21916=CARTESIAN_POINT('',(10.438768543395,1.,8.));
#21917=CARTESIAN_POINT('',(10.3045943951691,-1.,8.));
#21918=CARTESIAN_POINT('Origin',(10.1408077897493,-1.,8.45));
#21919=CARTESIAN_POINT('',(10.1408077897493,-1.,8.45));
#21920=CARTESIAN_POINT('',(10.3045943951691,-1.,8.));
#21921=CARTESIAN_POINT('',(10.1408077897493,1.,8.45));
#21922=CARTESIAN_POINT('',(10.3045943951691,1.,8.));
#21923=CARTESIAN_POINT('',(10.1408077897493,-1.,8.45));
#21924=CARTESIAN_POINT('Origin',(9.97423661809681,-1.,8.45));
#21925=CARTESIAN_POINT('',(9.97423661809681,-1.,8.45));
#21926=CARTESIAN_POINT('',(10.1408077897493,-1.,8.45));
#21927=CARTESIAN_POINT('',(9.97423661809681,1.,8.45));
#21928=CARTESIAN_POINT('',(10.1408077897493,1.,8.45));
#21929=CARTESIAN_POINT('',(9.97423661809681,-1.,8.45));
#21930=CARTESIAN_POINT('Origin',(9.81045001267702,-1.,8.));
#21931=CARTESIAN_POINT('',(9.81045001267702,-1.,8.));
#21932=CARTESIAN_POINT('',(9.97423661809681,-1.,8.45));
#21933=CARTESIAN_POINT('',(9.81045001267702,1.,8.));
#21934=CARTESIAN_POINT('',(9.97423661809681,1.,8.45));
#21935=CARTESIAN_POINT('',(9.81045001267702,-1.,8.));
#21936=CARTESIAN_POINT('Origin',(9.67627586445114,-1.,8.));
#21937=CARTESIAN_POINT('',(9.67627586445114,-1.,8.));
#21938=CARTESIAN_POINT('',(9.81045001267702,-1.,8.));
#21939=CARTESIAN_POINT('',(9.67627586445114,1.,8.));
#21940=CARTESIAN_POINT('',(9.81045001267702,1.,8.));
#21941=CARTESIAN_POINT('',(9.67627586445114,-1.,8.));
#21942=CARTESIAN_POINT('Origin',(9.51248925903135,-1.,8.45));
#21943=CARTESIAN_POINT('',(9.51248925903135,-1.,8.45));
#21944=CARTESIAN_POINT('',(9.67627586445114,-1.,8.));
#21945=CARTESIAN_POINT('',(9.51248925903135,1.,8.45));
#21946=CARTESIAN_POINT('',(9.67627586445114,1.,8.));
#21947=CARTESIAN_POINT('',(9.51248925903135,-1.,8.45));
#21948=CARTESIAN_POINT('Origin',(9.34591808737885,-1.,8.45));
#21949=CARTESIAN_POINT('',(9.34591808737885,-1.,8.45));
#21950=CARTESIAN_POINT('',(9.51248925903135,-1.,8.45));
#21951=CARTESIAN_POINT('',(9.34591808737885,1.,8.45));
#21952=CARTESIAN_POINT('',(9.51248925903135,1.,8.45));
#21953=CARTESIAN_POINT('',(9.34591808737885,-1.,8.45));
#21954=CARTESIAN_POINT('Origin',(9.18213148195906,-1.,8.));
#21955=CARTESIAN_POINT('',(9.18213148195906,-1.,8.));
#21956=CARTESIAN_POINT('',(9.34591808737885,-1.,8.45));
#21957=CARTESIAN_POINT('',(9.18213148195906,1.,8.));
#21958=CARTESIAN_POINT('',(9.34591808737885,1.,8.45));
#21959=CARTESIAN_POINT('',(9.18213148195906,-1.,8.));
#21960=CARTESIAN_POINT('Origin',(9.04795733373319,-1.,8.));
#21961=CARTESIAN_POINT('',(9.04795733373319,-1.,8.));
#21962=CARTESIAN_POINT('',(9.18213148195906,-1.,8.));
#21963=CARTESIAN_POINT('',(9.04795733373319,1.,8.));
#21964=CARTESIAN_POINT('',(9.18213148195906,1.,8.));
#21965=CARTESIAN_POINT('',(9.04795733373319,-1.,8.));
#21966=CARTESIAN_POINT('Origin',(8.88417072831339,-1.,8.45));
#21967=CARTESIAN_POINT('',(8.88417072831339,-1.,8.45));
#21968=CARTESIAN_POINT('',(9.04795733373319,-1.,8.));
#21969=CARTESIAN_POINT('',(8.88417072831339,1.,8.45));
#21970=CARTESIAN_POINT('',(9.04795733373319,1.,8.));
#21971=CARTESIAN_POINT('',(8.88417072831339,-1.,8.45));
#21972=CARTESIAN_POINT('Origin',(8.7175995566609,-1.,8.45));
#21973=CARTESIAN_POINT('',(8.7175995566609,-1.,8.45));
#21974=CARTESIAN_POINT('',(8.88417072831339,-1.,8.45));
#21975=CARTESIAN_POINT('',(8.7175995566609,1.,8.45));
#21976=CARTESIAN_POINT('',(8.88417072831339,1.,8.45));
#21977=CARTESIAN_POINT('',(8.7175995566609,-1.,8.45));
#21978=CARTESIAN_POINT('Origin',(8.5538129512411,-1.,8.));
#21979=CARTESIAN_POINT('',(8.5538129512411,-1.,8.));
#21980=CARTESIAN_POINT('',(8.7175995566609,-1.,8.45));
#21981=CARTESIAN_POINT('',(8.5538129512411,1.,8.));
#21982=CARTESIAN_POINT('',(8.7175995566609,1.,8.45));
#21983=CARTESIAN_POINT('',(8.5538129512411,-1.,8.));
#21984=CARTESIAN_POINT('Origin',(8.41963880301523,-1.,8.));
#21985=CARTESIAN_POINT('',(8.41963880301523,-1.,8.));
#21986=CARTESIAN_POINT('',(8.5538129512411,-1.,8.));
#21987=CARTESIAN_POINT('',(8.41963880301523,1.,8.));
#21988=CARTESIAN_POINT('',(8.5538129512411,1.,8.));
#21989=CARTESIAN_POINT('',(8.41963880301523,-1.,8.));
#21990=CARTESIAN_POINT('Origin',(8.25585219759544,-1.,8.45));
#21991=CARTESIAN_POINT('',(8.25585219759544,-1.,8.45));
#21992=CARTESIAN_POINT('',(8.41963880301523,-1.,8.));
#21993=CARTESIAN_POINT('',(8.25585219759544,1.,8.45));
#21994=CARTESIAN_POINT('',(8.41963880301523,1.,8.));
#21995=CARTESIAN_POINT('',(8.25585219759544,-1.,8.45));
#21996=CARTESIAN_POINT('Origin',(8.08928102594294,-1.,8.45));
#21997=CARTESIAN_POINT('',(8.08928102594294,-1.,8.45));
#21998=CARTESIAN_POINT('',(8.25585219759544,-1.,8.45));
#21999=CARTESIAN_POINT('',(8.08928102594294,1.,8.45));
#22000=CARTESIAN_POINT('',(8.25585219759544,1.,8.45));
#22001=CARTESIAN_POINT('',(8.08928102594294,-1.,8.45));
#22002=CARTESIAN_POINT('Origin',(7.92549442052315,-1.,8.));
#22003=CARTESIAN_POINT('',(7.92549442052315,-1.,8.));
#22004=CARTESIAN_POINT('',(8.08928102594294,-1.,8.45));
#22005=CARTESIAN_POINT('',(7.92549442052315,1.,8.));
#22006=CARTESIAN_POINT('',(8.08928102594294,1.,8.45));
#22007=CARTESIAN_POINT('',(7.92549442052315,-1.,8.));
#22008=CARTESIAN_POINT('Origin',(7.79132027229727,-1.,8.));
#22009=CARTESIAN_POINT('',(7.79132027229727,-1.,8.));
#22010=CARTESIAN_POINT('',(7.92549442052315,-1.,8.));
#22011=CARTESIAN_POINT('',(7.79132027229727,1.,8.));
#22012=CARTESIAN_POINT('',(7.92549442052315,1.,8.));
#22013=CARTESIAN_POINT('',(7.79132027229727,-1.,8.));
#22014=CARTESIAN_POINT('Origin',(7.62753366687748,-1.,8.45));
#22015=CARTESIAN_POINT('',(7.62753366687748,-1.,8.45));
#22016=CARTESIAN_POINT('',(7.79132027229727,-1.,8.));
#22017=CARTESIAN_POINT('',(7.62753366687748,1.,8.45));
#22018=CARTESIAN_POINT('',(7.79132027229727,1.,8.));
#22019=CARTESIAN_POINT('',(7.62753366687748,-1.,8.45));
#22020=CARTESIAN_POINT('Origin',(7.46096249522498,-1.,8.45));
#22021=CARTESIAN_POINT('',(7.46096249522498,-1.,8.45));
#22022=CARTESIAN_POINT('',(7.62753366687748,-1.,8.45));
#22023=CARTESIAN_POINT('',(7.46096249522498,1.,8.45));
#22024=CARTESIAN_POINT('',(7.62753366687748,1.,8.45));
#22025=CARTESIAN_POINT('',(7.46096249522498,-1.,8.45));
#22026=CARTESIAN_POINT('Origin',(7.29717588980519,-1.,8.));
#22027=CARTESIAN_POINT('',(7.29717588980519,-1.,8.));
#22028=CARTESIAN_POINT('',(7.46096249522498,-1.,8.45));
#22029=CARTESIAN_POINT('',(7.29717588980519,1.,8.));
#22030=CARTESIAN_POINT('',(7.46096249522498,1.,8.45));
#22031=CARTESIAN_POINT('',(7.29717588980519,-1.,8.));
#22032=CARTESIAN_POINT('Origin',(7.16300174157931,-1.,8.));
#22033=CARTESIAN_POINT('',(7.16300174157931,-1.,8.));
#22034=CARTESIAN_POINT('',(7.29717588980519,-1.,8.));
#22035=CARTESIAN_POINT('',(7.16300174157931,1.,8.));
#22036=CARTESIAN_POINT('',(7.29717588980519,1.,8.));
#22037=CARTESIAN_POINT('',(7.16300174157931,-1.,8.));
#22038=CARTESIAN_POINT('Origin',(6.99921513615952,-1.,8.45));
#22039=CARTESIAN_POINT('',(6.99921513615952,-1.,8.45));
#22040=CARTESIAN_POINT('',(7.16300174157931,-1.,8.));
#22041=CARTESIAN_POINT('',(6.99921513615952,1.,8.45));
#22042=CARTESIAN_POINT('',(7.16300174157931,1.,8.));
#22043=CARTESIAN_POINT('',(6.99921513615952,-1.,8.45));
#22044=CARTESIAN_POINT('Origin',(6.83264396450702,-1.,8.45));
#22045=CARTESIAN_POINT('',(6.83264396450702,-1.,8.45));
#22046=CARTESIAN_POINT('',(6.99921513615952,-1.,8.45));
#22047=CARTESIAN_POINT('',(6.83264396450702,1.,8.45));
#22048=CARTESIAN_POINT('',(6.99921513615952,1.,8.45));
#22049=CARTESIAN_POINT('',(6.83264396450702,-1.,8.45));
#22050=CARTESIAN_POINT('Origin',(6.66885735908723,-1.,8.));
#22051=CARTESIAN_POINT('',(6.66885735908723,-1.,8.));
#22052=CARTESIAN_POINT('',(6.83264396450702,-1.,8.45));
#22053=CARTESIAN_POINT('',(6.66885735908723,1.,8.));
#22054=CARTESIAN_POINT('',(6.83264396450702,1.,8.45));
#22055=CARTESIAN_POINT('',(6.66885735908723,-1.,8.));
#22056=CARTESIAN_POINT('Origin',(6.53468321086135,-1.,8.));
#22057=CARTESIAN_POINT('',(6.53468321086135,-1.,8.));
#22058=CARTESIAN_POINT('',(6.66885735908723,-1.,8.));
#22059=CARTESIAN_POINT('',(6.53468321086135,1.,8.));
#22060=CARTESIAN_POINT('',(6.66885735908723,1.,8.));
#22061=CARTESIAN_POINT('',(6.53468321086135,-1.,8.));
#22062=CARTESIAN_POINT('Origin',(6.37089660544156,-1.,8.45));
#22063=CARTESIAN_POINT('',(6.37089660544156,-1.,8.45));
#22064=CARTESIAN_POINT('',(6.53468321086135,-1.,8.));
#22065=CARTESIAN_POINT('',(6.37089660544156,1.,8.45));
#22066=CARTESIAN_POINT('',(6.53468321086135,1.,8.));
#22067=CARTESIAN_POINT('',(6.37089660544156,-1.,8.45));
#22068=CARTESIAN_POINT('Origin',(6.20432543378906,-1.,8.45));
#22069=CARTESIAN_POINT('',(6.20432543378906,-1.,8.45));
#22070=CARTESIAN_POINT('',(6.37089660544156,-1.,8.45));
#22071=CARTESIAN_POINT('',(6.20432543378906,1.,8.45));
#22072=CARTESIAN_POINT('',(6.37089660544156,1.,8.45));
#22073=CARTESIAN_POINT('',(6.20432543378906,-1.,8.45));
#22074=CARTESIAN_POINT('Origin',(6.04053882836927,-1.,8.));
#22075=CARTESIAN_POINT('',(6.04053882836927,-1.,8.));
#22076=CARTESIAN_POINT('',(6.20432543378906,-1.,8.45));
#22077=CARTESIAN_POINT('',(6.04053882836927,1.,8.));
#22078=CARTESIAN_POINT('',(6.20432543378906,1.,8.45));
#22079=CARTESIAN_POINT('',(6.04053882836927,-1.,8.));
#22080=CARTESIAN_POINT('Origin',(5.90636468014339,-1.,8.));
#22081=CARTESIAN_POINT('',(5.90636468014339,-1.,8.));
#22082=CARTESIAN_POINT('',(6.04053882836927,-1.,8.));
#22083=CARTESIAN_POINT('',(5.90636468014339,1.,8.));
#22084=CARTESIAN_POINT('',(6.04053882836927,1.,8.));
#22085=CARTESIAN_POINT('',(5.90636468014339,-1.,8.));
#22086=CARTESIAN_POINT('Origin',(5.7425780747236,-1.,8.45));
#22087=CARTESIAN_POINT('',(5.7425780747236,-1.,8.45));
#22088=CARTESIAN_POINT('',(5.90636468014339,-1.,8.));
#22089=CARTESIAN_POINT('',(5.7425780747236,1.,8.45));
#22090=CARTESIAN_POINT('',(5.90636468014339,1.,8.));
#22091=CARTESIAN_POINT('',(5.7425780747236,-1.,8.45));
#22092=CARTESIAN_POINT('Origin',(5.5760069030711,-1.,8.45));
#22093=CARTESIAN_POINT('',(5.5760069030711,-1.,8.45));
#22094=CARTESIAN_POINT('',(5.7425780747236,-1.,8.45));
#22095=CARTESIAN_POINT('',(5.5760069030711,1.,8.45));
#22096=CARTESIAN_POINT('',(5.7425780747236,1.,8.45));
#22097=CARTESIAN_POINT('',(5.5760069030711,-1.,8.45));
#22098=CARTESIAN_POINT('Origin',(5.41222029765131,-1.,8.));
#22099=CARTESIAN_POINT('',(5.41222029765131,-1.,8.));
#22100=CARTESIAN_POINT('',(5.5760069030711,-1.,8.45));
#22101=CARTESIAN_POINT('',(5.41222029765131,1.,8.));
#22102=CARTESIAN_POINT('',(5.5760069030711,1.,8.45));
#22103=CARTESIAN_POINT('',(5.41222029765131,-1.,8.));
#22104=CARTESIAN_POINT('Origin',(5.27804614942543,-1.,8.));
#22105=CARTESIAN_POINT('',(5.27804614942543,-1.,8.));
#22106=CARTESIAN_POINT('',(5.41222029765131,-1.,8.));
#22107=CARTESIAN_POINT('',(5.27804614942543,1.,8.));
#22108=CARTESIAN_POINT('',(5.41222029765131,1.,8.));
#22109=CARTESIAN_POINT('',(5.27804614942543,-1.,8.));
#22110=CARTESIAN_POINT('Origin',(5.11425954400564,-1.,8.45));
#22111=CARTESIAN_POINT('',(5.11425954400564,-1.,8.45));
#22112=CARTESIAN_POINT('',(5.27804614942543,-1.,8.));
#22113=CARTESIAN_POINT('',(5.11425954400564,1.,8.45));
#22114=CARTESIAN_POINT('',(5.27804614942543,1.,8.));
#22115=CARTESIAN_POINT('',(5.11425954400564,-1.,8.45));
#22116=CARTESIAN_POINT('Origin',(4.94768837235314,-1.,8.45));
#22117=CARTESIAN_POINT('',(4.94768837235314,-1.,8.45));
#22118=CARTESIAN_POINT('',(5.11425954400564,-1.,8.45));
#22119=CARTESIAN_POINT('',(4.94768837235314,1.,8.45));
#22120=CARTESIAN_POINT('',(5.11425954400564,1.,8.45));
#22121=CARTESIAN_POINT('',(4.94768837235314,-1.,8.45));
#22122=CARTESIAN_POINT('Origin',(4.78390176693335,-1.,8.));
#22123=CARTESIAN_POINT('',(4.78390176693335,-1.,8.));
#22124=CARTESIAN_POINT('',(4.94768837235314,-1.,8.45));
#22125=CARTESIAN_POINT('',(4.78390176693335,1.,8.));
#22126=CARTESIAN_POINT('',(4.94768837235314,1.,8.45));
#22127=CARTESIAN_POINT('',(4.78390176693335,-1.,8.));
#22128=CARTESIAN_POINT('Origin',(4.64972761870748,-1.,8.));
#22129=CARTESIAN_POINT('',(4.64972761870748,-1.,8.));
#22130=CARTESIAN_POINT('',(4.78390176693335,-1.,8.));
#22131=CARTESIAN_POINT('',(4.64972761870748,1.,8.));
#22132=CARTESIAN_POINT('',(4.78390176693335,1.,8.));
#22133=CARTESIAN_POINT('',(4.64972761870748,-1.,8.));
#22134=CARTESIAN_POINT('Origin',(4.48594101328768,-1.,8.45));
#22135=CARTESIAN_POINT('',(4.48594101328768,-1.,8.45));
#22136=CARTESIAN_POINT('',(4.64972761870748,-1.,8.));
#22137=CARTESIAN_POINT('',(4.48594101328768,1.,8.45));
#22138=CARTESIAN_POINT('',(4.64972761870748,1.,8.));
#22139=CARTESIAN_POINT('',(4.48594101328768,-1.,8.45));
#22140=CARTESIAN_POINT('Origin',(4.31936984163519,-1.,8.45));
#22141=CARTESIAN_POINT('',(4.31936984163519,-1.,8.45));
#22142=CARTESIAN_POINT('',(4.48594101328768,-1.,8.45));
#22143=CARTESIAN_POINT('',(4.31936984163519,1.,8.45));
#22144=CARTESIAN_POINT('',(4.48594101328768,1.,8.45));
#22145=CARTESIAN_POINT('',(4.31936984163519,-1.,8.45));
#22146=CARTESIAN_POINT('Origin',(4.15558323621539,-1.,8.));
#22147=CARTESIAN_POINT('',(4.15558323621539,-1.,8.));
#22148=CARTESIAN_POINT('',(4.31936984163519,-1.,8.45));
#22149=CARTESIAN_POINT('',(4.15558323621539,1.,8.));
#22150=CARTESIAN_POINT('',(4.31936984163519,1.,8.45));
#22151=CARTESIAN_POINT('',(4.15558323621539,-1.,8.));
#22152=CARTESIAN_POINT('Origin',(4.02140908798952,-1.,8.));
#22153=CARTESIAN_POINT('',(4.02140908798952,-1.,8.));
#22154=CARTESIAN_POINT('',(4.15558323621539,-1.,8.));
#22155=CARTESIAN_POINT('',(4.02140908798952,1.,8.));
#22156=CARTESIAN_POINT('',(4.15558323621539,1.,8.));
#22157=CARTESIAN_POINT('',(4.02140908798952,-1.,8.));
#22158=CARTESIAN_POINT('Origin',(3.85762248256973,-1.,8.45));
#22159=CARTESIAN_POINT('',(3.85762248256973,-1.,8.45));
#22160=CARTESIAN_POINT('',(4.02140908798952,-1.,8.));
#22161=CARTESIAN_POINT('',(3.85762248256973,1.,8.45));
#22162=CARTESIAN_POINT('',(4.02140908798952,1.,8.));
#22163=CARTESIAN_POINT('',(3.85762248256973,-1.,8.45));
#22164=CARTESIAN_POINT('Origin',(3.69105131091723,-1.,8.45));
#22165=CARTESIAN_POINT('',(3.69105131091723,-1.,8.45));
#22166=CARTESIAN_POINT('',(3.85762248256973,-1.,8.45));
#22167=CARTESIAN_POINT('',(3.69105131091723,1.,8.45));
#22168=CARTESIAN_POINT('',(3.85762248256973,1.,8.45));
#22169=CARTESIAN_POINT('',(3.69105131091723,-1.,8.45));
#22170=CARTESIAN_POINT('Origin',(3.52726470549744,-1.,8.));
#22171=CARTESIAN_POINT('',(3.52726470549744,-1.,8.));
#22172=CARTESIAN_POINT('',(3.69105131091723,-1.,8.45));
#22173=CARTESIAN_POINT('',(3.52726470549744,1.,8.));
#22174=CARTESIAN_POINT('',(3.69105131091723,1.,8.45));
#22175=CARTESIAN_POINT('',(3.52726470549744,-1.,8.));
#22176=CARTESIAN_POINT('Origin',(3.39309055727156,-1.,8.));
#22177=CARTESIAN_POINT('',(3.39309055727156,-1.,8.));
#22178=CARTESIAN_POINT('',(3.52726470549744,-1.,8.));
#22179=CARTESIAN_POINT('',(3.39309055727156,1.,8.));
#22180=CARTESIAN_POINT('',(3.52726470549744,1.,8.));
#22181=CARTESIAN_POINT('',(3.39309055727156,-1.,8.));
#22182=CARTESIAN_POINT('Origin',(3.22930395185177,-1.,8.45));
#22183=CARTESIAN_POINT('',(3.22930395185177,-1.,8.45));
#22184=CARTESIAN_POINT('',(3.39309055727156,-1.,8.));
#22185=CARTESIAN_POINT('',(3.22930395185177,1.,8.45));
#22186=CARTESIAN_POINT('',(3.39309055727156,1.,8.));
#22187=CARTESIAN_POINT('',(3.22930395185177,-1.,8.45));
#22188=CARTESIAN_POINT('Origin',(3.06273278019927,-1.,8.45));
#22189=CARTESIAN_POINT('',(3.06273278019927,-1.,8.45));
#22190=CARTESIAN_POINT('',(3.22930395185177,-1.,8.45));
#22191=CARTESIAN_POINT('',(3.06273278019927,1.,8.45));
#22192=CARTESIAN_POINT('',(3.22930395185177,1.,8.45));
#22193=CARTESIAN_POINT('',(3.06273278019927,-1.,8.45));
#22194=CARTESIAN_POINT('Origin',(2.89894617477948,-1.,8.));
#22195=CARTESIAN_POINT('',(2.89894617477948,-1.,8.));
#22196=CARTESIAN_POINT('',(3.06273278019927,-1.,8.45));
#22197=CARTESIAN_POINT('',(2.89894617477948,1.,8.));
#22198=CARTESIAN_POINT('',(3.06273278019927,1.,8.45));
#22199=CARTESIAN_POINT('',(2.89894617477948,-1.,8.));
#22200=CARTESIAN_POINT('Origin',(2.7647720265536,-1.,8.));
#22201=CARTESIAN_POINT('',(2.7647720265536,-1.,8.));
#22202=CARTESIAN_POINT('',(2.89894617477948,-1.,8.));
#22203=CARTESIAN_POINT('',(2.7647720265536,1.,8.));
#22204=CARTESIAN_POINT('',(2.89894617477948,1.,8.));
#22205=CARTESIAN_POINT('',(2.7647720265536,-1.,8.));
#22206=CARTESIAN_POINT('Origin',(2.60098542113381,-1.,8.45));
#22207=CARTESIAN_POINT('',(2.60098542113381,-1.,8.45));
#22208=CARTESIAN_POINT('',(2.7647720265536,-1.,8.));
#22209=CARTESIAN_POINT('',(2.60098542113381,1.,8.45));
#22210=CARTESIAN_POINT('',(2.7647720265536,1.,8.));
#22211=CARTESIAN_POINT('',(2.60098542113381,-1.,8.45));
#22212=CARTESIAN_POINT('Origin',(2.43441424948131,-1.,8.45));
#22213=CARTESIAN_POINT('',(2.43441424948131,-1.,8.45));
#22214=CARTESIAN_POINT('',(2.60098542113381,-1.,8.45));
#22215=CARTESIAN_POINT('',(2.43441424948131,1.,8.45));
#22216=CARTESIAN_POINT('',(2.60098542113381,1.,8.45));
#22217=CARTESIAN_POINT('',(2.43441424948131,-1.,8.45));
#22218=CARTESIAN_POINT('Origin',(2.27062764406152,-1.,8.));
#22219=CARTESIAN_POINT('',(2.27062764406152,-1.,8.));
#22220=CARTESIAN_POINT('',(2.43441424948131,-1.,8.45));
#22221=CARTESIAN_POINT('',(2.27062764406152,1.,8.));
#22222=CARTESIAN_POINT('',(2.43441424948131,1.,8.45));
#22223=CARTESIAN_POINT('',(2.27062764406152,-1.,8.));
#22224=CARTESIAN_POINT('Origin',(2.13645349583564,-1.,8.));
#22225=CARTESIAN_POINT('',(2.13645349583564,-1.,8.));
#22226=CARTESIAN_POINT('',(2.27062764406152,-1.,8.));
#22227=CARTESIAN_POINT('',(2.13645349583564,1.,8.));
#22228=CARTESIAN_POINT('',(2.27062764406152,1.,8.));
#22229=CARTESIAN_POINT('',(2.13645349583564,-1.,8.));
#22230=CARTESIAN_POINT('Origin',(1.97266689041585,-1.,8.45));
#22231=CARTESIAN_POINT('',(1.97266689041585,-1.,8.45));
#22232=CARTESIAN_POINT('',(2.13645349583564,-1.,8.));
#22233=CARTESIAN_POINT('',(1.97266689041585,1.,8.45));
#22234=CARTESIAN_POINT('',(2.13645349583564,1.,8.));
#22235=CARTESIAN_POINT('',(1.97266689041585,-1.,8.45));
#22236=CARTESIAN_POINT('Origin',(1.80609571876335,-1.,8.45));
#22237=CARTESIAN_POINT('',(1.80609571876335,-1.,8.45));
#22238=CARTESIAN_POINT('',(1.97266689041585,-1.,8.45));
#22239=CARTESIAN_POINT('',(1.80609571876335,1.,8.45));
#22240=CARTESIAN_POINT('',(1.97266689041585,1.,8.45));
#22241=CARTESIAN_POINT('',(1.80609571876335,-1.,8.45));
#22242=CARTESIAN_POINT('Origin',(1.64230911334356,-1.,8.));
#22243=CARTESIAN_POINT('',(1.64230911334356,-1.,8.));
#22244=CARTESIAN_POINT('',(1.80609571876335,-1.,8.45));
#22245=CARTESIAN_POINT('',(1.64230911334356,1.,8.));
#22246=CARTESIAN_POINT('',(1.80609571876335,1.,8.45));
#22247=CARTESIAN_POINT('',(1.64230911334356,-1.,8.));
#22248=CARTESIAN_POINT('Origin',(1.,-1.,8.));
#22249=CARTESIAN_POINT('',(1.64230911334356,-1.,8.));
#22250=CARTESIAN_POINT('',(1.64230911334356,1.,8.));
#22251=CARTESIAN_POINT('Origin',(11.,1.,7.725));
#22252=CARTESIAN_POINT('Origin',(11.,-1.,7.725));
#34774=UNCERTAINTY_MEASURE_WITH_UNIT(LENGTH_MEASURE(0.001),#34852,
'DISTANCE_ACCURACY_VALUE',
'Maximum model space distance between geometric entities at asserted c
onnectivities');
#34797=UNCERTAINTY_MEASURE_WITH_UNIT(LENGTH_MEASURE(0.001),#34852,
'DISTANCE_ACCURACY_VALUE',
'Maximum model space distance between geometric entities at asserted c
onnectivities');
#34828=(
GEOMETRIC_REPRESENTATION_CONTEXT(3)
GLOBAL_UNCERTAINTY_ASSIGNED_CONTEXT((#34774))
GLOBAL_UNIT_ASSIGNED_CONTEXT((#34852,#34854,#34855))
REPRESENTATION_CONTEXT('','3D')
);
#34851=(
GEOMETRIC_REPRESENTATION_CONTEXT(3)
GLOBAL_UNCERTAINTY_ASSIGNED_CONTEXT((#34797))
GLOBAL_UNIT_ASSIGNED_CONTEXT((#34852,#34854,#34855))
REPRESENTATION_CONTEXT('','3D')
);
#34852=(
LENGTH_UNIT()
NAMED_UNIT(*)
SI_UNIT(.CENTI.,.METRE.)
);
#34854=(
NAMED_UNIT(*)
PLANE_ANGLE_UNIT()
SI_UNIT($,.RADIAN.)
);
#34855=(
NAMED_UNIT(*)
SI_UNIT($,.STERADIAN.)
SOLID_ANGLE_UNIT()
);
#34886=SHAPE_DEFINITION_REPRESENTATION(#34944,#35103);
#34944=PRODUCT_DEFINITION_SHAPE('',$,#35157);
#35103=SHAPE_REPRESENTATION('',(#14962),#34828);
#35126=PRODUCT_DEFINITION_CONTEXT('part definition',#35287,'design');
#35157=PRODUCT_DEFINITION('Module 2 rack','Module 2 rack',#35210,#35126);
#35210=PRODUCT_DEFINITION_FORMATION('',$,#35319);
#35287=APPLICATION_CONTEXT(
'Core Data for Automotive Mechanical Design Process');
#35288=PRODUCT_CONTEXT('part definition',#35287,'mechanical');
#35319=PRODUCT('Module 2 rack','Module 2 rack','Module 2 rack',(#35288));
#35391=COLOUR_RGB('Light Blue',0.38,0.62,0.78);
#35392=FILL_AREA_STYLE_COLOUR('',#35391);
#35393=FILL_AREA_STYLE('',(#35392));
#35394=SURFACE_STYLE_FILL_AREA(#35393);
#35395=SURFACE_SIDE_STYLE('',(#35394));
#35396=SURFACE_STYLE_USAGE(.BOTH.,#35395);
#35397=PRESENTATION_STYLE_ASSIGNMENT((#35396));
ENDSEC;
END-ISO-10303-21;
